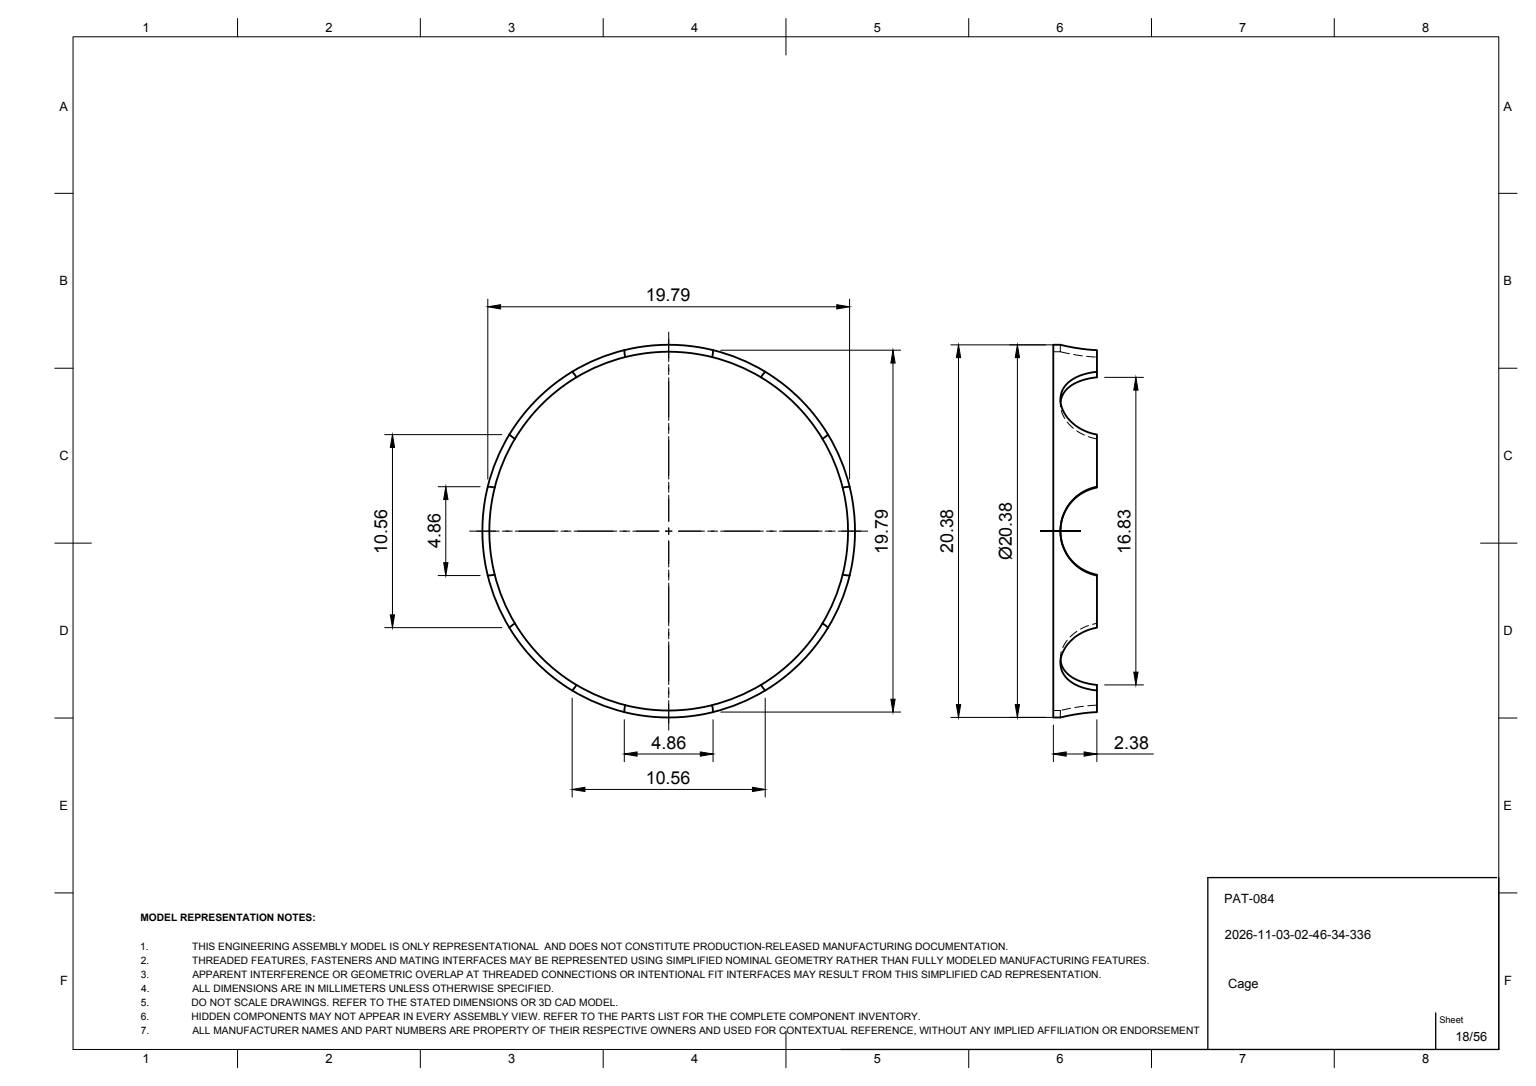
ISO-10303-21;
HEADER;
/* Generated by software containing ST-Developer
 * from STEP Tools, Inc. (www.steptools.com) 
 */

FILE_DESCRIPTION(
/* description */ ('Quick-return (Whitworth) mechanism'),
/* implementation_level */ '2;1');

FILE_NAME(
/* name */ 'Cage.step',
/* time_stamp */ '2026-10-28T03:25:57-07:00',
/* author */ (''),
/* organization */ (''),
/* preprocessor_version */ 'ST-DEVELOPER v20.2',
/* originating_system */ 'Autodesk Translation Framework v15.17.0.0',
/* authorisation */ '');

FILE_SCHEMA (('AUTOMOTIVE_DESIGN { 1 0 10303 214 3 1 1 }'));
ENDSEC;

DATA;
#10=MECHANICAL_DESIGN_GEOMETRIC_PRESENTATION_REPRESENTATION('',(#508),#14878);
#341=SPHERICAL_SURFACE('',#8767,0.247676);
#342=SPHERICAL_SURFACE('',#8783,0.247676);
#343=SPHERICAL_SURFACE('',#8788,0.247676);
#344=SPHERICAL_SURFACE('',#8793,0.247676);
#345=SPHERICAL_SURFACE('',#8798,0.247676);
#346=SPHERICAL_SURFACE('',#8803,0.247676);
#347=SPHERICAL_SURFACE('',#8808,0.247676);
#348=SPHERICAL_SURFACE('',#8816,0.247676);
#374=B_SPLINE_CURVE_WITH_KNOTS('',3,(#12898,#12899,#12900,#12901,#12902,
#12903,#12904,#12905,#12906,#12907,#12908,#12909,#12910,#12911,#12912,#12913,
#12914,#12915,#12916,#12917,#12918,#12919),.UNSPECIFIED.,.F.,.F.,(4,2,2,
2,2,2,2,2,2,2,4),(0.0473477652366656,0.126350602536658,0.189525903804987,
0.252701205073317,0.313298422430275,0.373895639787233,0.434492857144191,
0.495090074501149,0.558265375769478,0.621440677037807,0.7004435143378),
 .UNSPECIFIED.);
#375=B_SPLINE_CURVE_WITH_KNOTS('',3,(#12923,#12924,#12925,#12926,#12927,
#12928,#12929,#12930,#12931,#12932,#12933,#12934,#12935,#12936,#12937,#12938,
#12939,#12940,#12941,#12942,#12943,#12944),.UNSPECIFIED.,.F.,.F.,(4,2,2,
2,2,2,2,2,2,2,4),(0.0464897534940957,0.0852567806515119,0.170513561303024,
0.246687263103517,0.308657850341199,0.370628437578881,0.432599024816563,
0.494569612054245,0.570743313854739,0.656000094506251,0.694767121663666),
 .UNSPECIFIED.);
#376=B_SPLINE_CURVE_WITH_KNOTS('',3,(#12950,#12951,#12952,#12953,#12954,
#12955,#12956,#12957,#12958,#12959,#12960,#12961,#12962,#12963,#12964,#12965,
#12966,#12967,#12968,#12969,#12970,#12971),.UNSPECIFIED.,.F.,.F.,(4,2,2,
2,2,2,2,2,2,2,4),(0.0464897534940957,0.0852567806515118,0.170513561303024,
0.246687263103517,0.308657850341199,0.370628437578881,0.432599024816563,
0.494569612054245,0.570743313854738,0.65600009450625,0.694767121663666),
 .UNSPECIFIED.);
#377=B_SPLINE_CURVE_WITH_KNOTS('',3,(#12975,#12976,#12977,#12978,#12979,
#12980,#12981,#12982,#12983,#12984,#12985,#12986,#12987,#12988,#12989,#12990,
#12991,#12992,#12993,#12994,#12995,#12996),.UNSPECIFIED.,.F.,.F.,(4,2,2,
2,2,2,2,2,2,2,4),(0.0464897534940957,0.0852567806515119,0.170513561303024,
0.246687263103517,0.308657850341199,0.370628437578881,0.432599024816563,
0.494569612054245,0.570743313854739,0.656000094506251,0.694767121663666),
 .UNSPECIFIED.);
#378=B_SPLINE_CURVE_WITH_KNOTS('',3,(#13000,#13001,#13002,#13003,#13004,
#13005,#13006,#13007,#13008,#13009,#13010,#13011),.UNSPECIFIED.,.F.,.F.,
(4,2,2,2,2,4),(0.0464897534940957,0.0852567806515119,0.170513561303024,
0.246687263103517,0.308657850341199,0.370628437578881),.UNSPECIFIED.);
#379=B_SPLINE_CURVE_WITH_KNOTS('',3,(#13016,#13017,#13018,#13019,#13020,
#13021,#13022,#13023,#13024,#13025,#13026,#13027),.UNSPECIFIED.,.F.,.F.,
(4,2,2,2,2,4),(0.370628437578881,0.432599024816563,0.494569612054245,0.570743313854738,
0.65600009450625,0.694767121663666),.UNSPECIFIED.);
#380=B_SPLINE_CURVE_WITH_KNOTS('',3,(#13031,#13032,#13033,#13034,#13035,
#13036,#13037,#13038,#13039,#13040,#13041,#13042,#13043,#13044,#13045,#13046,
#13047,#13048,#13049,#13050,#13051,#13052),.UNSPECIFIED.,.F.,.F.,(4,2,2,
2,2,2,2,2,2,2,4),(0.0464897534940957,0.0852567806515121,0.170513561303024,
0.246687263103518,0.308657850341199,0.370628437578881,0.432599024816563,
0.494569612054245,0.570743313854738,0.65600009450625,0.694767121663666),
 .UNSPECIFIED.);
#381=B_SPLINE_CURVE_WITH_KNOTS('',3,(#13056,#13057,#13058,#13059,#13060,
#13061,#13062,#13063,#13064,#13065,#13066,#13067,#13068,#13069,#13070,#13071,
#13072,#13073,#13074,#13075,#13076,#13077),.UNSPECIFIED.,.F.,.F.,(4,2,2,
2,2,2,2,2,2,2,4),(0.0464897534940957,0.0852567806515119,0.170513561303024,
0.246687263103517,0.308657850341199,0.370628437578881,0.432599024816563,
0.494569612054245,0.570743313854738,0.65600009450625,0.694767121663667),
 .UNSPECIFIED.);
#382=B_SPLINE_CURVE_WITH_KNOTS('',3,(#13081,#13082,#13083,#13084,#13085,
#13086,#13087,#13088,#13089,#13090,#13091,#13092,#13093,#13094,#13095,#13096,
#13097,#13098,#13099,#13100,#13101,#13102),.UNSPECIFIED.,.F.,.F.,(4,2,2,
2,2,2,2,2,2,2,4),(0.0464897534940957,0.0852567806515119,0.170513561303024,
0.246687263103517,0.308657850341199,0.370628437578881,0.432599024816563,
0.494569612054245,0.570743313854738,0.65600009450625,0.694767121663666),
 .UNSPECIFIED.);
#383=B_SPLINE_CURVE_WITH_KNOTS('',3,(#13106,#13107,#13108,#13109,#13110,
#13111,#13112,#13113,#13114,#13115,#13116,#13117,#13118,#13119,#13120,#13121,
#13122,#13123,#13124,#13125,#13126,#13127),.UNSPECIFIED.,.F.,.F.,(4,2,2,
2,2,2,2,2,2,2,4),(0.0464897534940957,0.0852567806515119,0.170513561303024,
0.246687263103517,0.308657850341199,0.370628437578881,0.432599024816563,
0.494569612054245,0.570743313854739,0.656000094506251,0.694767121663667),
 .UNSPECIFIED.);
#384=B_SPLINE_CURVE_WITH_KNOTS('',3,(#13135,#13136,#13137,#13138,#13139,
#13140,#13141,#13142,#13143,#13144,#13145,#13146,#13147,#13148,#13149,#13150,
#13151,#13152,#13153,#13154,#13155,#13156),.UNSPECIFIED.,.F.,.F.,(4,2,2,
2,2,2,2,2,2,2,4),(0.0473477652366656,0.126350602536658,0.189525903804987,
0.252701205073316,0.313298422430274,0.373895639787232,0.434492857144191,
0.495090074501149,0.558265375769478,0.621440677037807,0.7004435143378),
 .UNSPECIFIED.);
#385=B_SPLINE_CURVE_WITH_KNOTS('',3,(#13164,#13165,#13166,#13167,#13168,
#13169,#13170,#13171,#13172,#13173,#13174,#13175,#13176,#13177,#13178,#13179,
#13180,#13181,#13182,#13183,#13184,#13185),.UNSPECIFIED.,.F.,.F.,(4,2,2,
2,2,2,2,2,2,2,4),(0.0473477652366656,0.126350602536658,0.189525903804987,
0.252701205073317,0.313298422430275,0.373895639787233,0.434492857144191,
0.495090074501149,0.558265375769478,0.621440677037807,0.7004435143378),
 .UNSPECIFIED.);
#386=B_SPLINE_CURVE_WITH_KNOTS('',3,(#13194,#13195,#13196,#13197,#13198,
#13199,#13200,#13201,#13202,#13203,#13204,#13205),.UNSPECIFIED.,.F.,.F.,
(4,2,2,2,2,4),(0.0473477652366656,0.126350602536658,0.189525903804987,0.252701205073316,
0.313298422430275,0.373895639787233),.UNSPECIFIED.);
#387=B_SPLINE_CURVE_WITH_KNOTS('',3,(#13207,#13208,#13209,#13210,#13211,
#13212,#13213,#13214,#13215,#13216,#13217,#13218),.UNSPECIFIED.,.F.,.F.,
(4,2,2,2,2,4),(0.373895639787233,0.434492857144191,0.495090074501149,0.558265375769478,
0.621440677037807,0.7004435143378),.UNSPECIFIED.);
#388=B_SPLINE_CURVE_WITH_KNOTS('',3,(#13225,#13226,#13227,#13228,#13229,
#13230,#13231,#13232,#13233,#13234,#13235,#13236,#13237,#13238,#13239,#13240,
#13241,#13242,#13243,#13244,#13245,#13246),.UNSPECIFIED.,.F.,.F.,(4,2,2,
2,2,2,2,2,2,2,4),(0.0473477652366656,0.126350602536658,0.189525903804987,
0.252701205073316,0.313298422430275,0.373895639787233,0.434492857144191,
0.495090074501149,0.558265375769478,0.621440677037807,0.7004435143378),
 .UNSPECIFIED.);
#389=B_SPLINE_CURVE_WITH_KNOTS('',3,(#13254,#13255,#13256,#13257,#13258,
#13259,#13260,#13261,#13262,#13263,#13264,#13265,#13266,#13267,#13268,#13269,
#13270,#13271,#13272,#13273,#13274,#13275),.UNSPECIFIED.,.F.,.F.,(4,2,2,
2,2,2,2,2,2,2,4),(0.0473477652366656,0.126350602536658,0.189525903804987,
0.252701205073317,0.313298422430275,0.373895639787233,0.434492857144191,
0.495090074501149,0.558265375769478,0.621440677037807,0.7004435143378),
 .UNSPECIFIED.);
#390=B_SPLINE_CURVE_WITH_KNOTS('',3,(#13283,#13284,#13285,#13286,#13287,
#13288,#13289,#13290,#13291,#13292,#13293,#13294,#13295,#13296,#13297,#13298,
#13299,#13300,#13301,#13302,#13303,#13304),.UNSPECIFIED.,.F.,.F.,(4,2,2,
2,2,2,2,2,2,2,4),(0.0473477652366656,0.126350602536658,0.189525903804987,
0.252701205073316,0.313298422430275,0.373895639787233,0.434492857144191,
0.495090074501149,0.558265375769478,0.621440677037807,0.7004435143378),
 .UNSPECIFIED.);
#391=B_SPLINE_CURVE_WITH_KNOTS('',3,(#13313,#13314,#13315,#13316,#13317,
#13318,#13319,#13320,#13321,#13322,#13323,#13324,#13325,#13326,#13327,#13328,
#13329,#13330,#13331,#13332,#13333,#13334),.UNSPECIFIED.,.F.,.F.,(4,2,2,
2,2,2,2,2,2,2,4),(0.0473477652366656,0.126350602536658,0.189525903804987,
0.252701205073317,0.313298422430275,0.373895639787233,0.434492857144191,
0.495090074501149,0.558265375769478,0.621440677037807,0.7004435143378),
 .UNSPECIFIED.);
#413=SHAPE_REPRESENTATION_RELATIONSHIP('SRR','None',#15082,#457);
#457=ADVANCED_BREP_SHAPE_REPRESENTATION('',(#560),#14839);
#508=STYLED_ITEM('',(#15406),#560);
#560=MANIFOLD_SOLID_BREP('Continuous crown cage',#7862);
#697=FACE_BOUND('',#1811,.T.);
#860=PLANE('',#8780);
#861=PLANE('',#8785);
#862=PLANE('',#8790);
#863=PLANE('',#8795);
#864=PLANE('',#8800);
#865=PLANE('',#8805);
#866=PLANE('',#8814);
#867=PLANE('',#8818);
#868=PLANE('',#8819);
#1221=FACE_OUTER_BOUND('',#1793,.T.);
#1222=FACE_OUTER_BOUND('',#1794,.T.);
#1223=FACE_OUTER_BOUND('',#1795,.T.);
#1224=FACE_OUTER_BOUND('',#1796,.T.);
#1225=FACE_OUTER_BOUND('',#1797,.T.);
#1226=FACE_OUTER_BOUND('',#1798,.T.);
#1227=FACE_OUTER_BOUND('',#1799,.T.);
#1228=FACE_OUTER_BOUND('',#1800,.T.);
#1229=FACE_OUTER_BOUND('',#1801,.T.);
#1230=FACE_OUTER_BOUND('',#1802,.T.);
#1231=FACE_OUTER_BOUND('',#1803,.T.);
#1232=FACE_OUTER_BOUND('',#1804,.T.);
#1233=FACE_OUTER_BOUND('',#1805,.T.);
#1234=FACE_OUTER_BOUND('',#1806,.T.);
#1235=FACE_OUTER_BOUND('',#1807,.T.);
#1236=FACE_OUTER_BOUND('',#1808,.T.);
#1237=FACE_OUTER_BOUND('',#1809,.T.);
#1238=FACE_OUTER_BOUND('',#1810,.T.);
#1239=FACE_OUTER_BOUND('',#1812,.T.);
#1793=EDGE_LOOP('',(#5998,#5999,#6000,#6001));
#1794=EDGE_LOOP('',(#6002,#6003,#6004,#6005,#6006,#6007,#6008,#6009,#6010,
#6011,#6012,#6013,#6014,#6015,#6016,#6017,#6018,#6019,#6020,#6021));
#1795=EDGE_LOOP('',(#6022,#6023,#6024,#6025));
#1796=EDGE_LOOP('',(#6026,#6027,#6028,#6029));
#1797=EDGE_LOOP('',(#6030,#6031,#6032,#6033));
#1798=EDGE_LOOP('',(#6034,#6035,#6036,#6037));
#1799=EDGE_LOOP('',(#6038,#6039,#6040,#6041));
#1800=EDGE_LOOP('',(#6042,#6043,#6044,#6045,#6046,#6047));
#1801=EDGE_LOOP('',(#6048,#6049,#6050,#6051));
#1802=EDGE_LOOP('',(#6052,#6053,#6054,#6055));
#1803=EDGE_LOOP('',(#6056,#6057,#6058,#6059));
#1804=EDGE_LOOP('',(#6060,#6061,#6062,#6063));
#1805=EDGE_LOOP('',(#6064,#6065,#6066,#6067));
#1806=EDGE_LOOP('',(#6068,#6069,#6070,#6071));
#1807=EDGE_LOOP('',(#6072,#6073,#6074,#6075,#6076,#6077,#6078,#6079,#6080,
#6081,#6082,#6083,#6084,#6085,#6086,#6087,#6088,#6089,#6090,#6091));
#1808=EDGE_LOOP('',(#6092,#6093,#6094,#6095));
#1809=EDGE_LOOP('',(#6096,#6097,#6098,#6099));
#1810=EDGE_LOOP('',(#6100));
#1811=EDGE_LOOP('',(#6101));
#1812=EDGE_LOOP('',(#6102,#6103,#6104,#6105));
#2336=LINE('',#13013,#2859);
#2337=LINE('',#13309,#2860);
#2859=VECTOR('',#10343,1.019052);
#2860=VECTOR('',#10420,0.980948);
#3410=CIRCLE('',#8768,0.243053047864041);
#3411=CIRCLE('',#8769,0.243053047864041);
#3412=CIRCLE('',#8771,1.019052);
#3413=CIRCLE('',#8772,1.019052);
#3414=CIRCLE('',#8773,1.019052);
#3415=CIRCLE('',#8774,1.019052);
#3416=CIRCLE('',#8775,1.019052);
#3417=CIRCLE('',#8776,1.019052);
#3418=CIRCLE('',#8777,1.019052);
#3419=CIRCLE('',#8778,1.019052);
#3420=CIRCLE('',#8779,1.019052);
#3421=CIRCLE('',#8781,0.980948);
#3422=CIRCLE('',#8782,0.243053047864041);
#3423=CIRCLE('',#8784,0.243053047864041);
#3424=CIRCLE('',#8786,0.980948);
#3425=CIRCLE('',#8787,0.243053047864041);
#3426=CIRCLE('',#8789,0.243053047864041);
#3427=CIRCLE('',#8791,0.980948);
#3428=CIRCLE('',#8792,0.243053047864041);
#3429=CIRCLE('',#8794,0.243053047864041);
#3430=CIRCLE('',#8796,0.980948);
#3431=CIRCLE('',#8797,0.243053047864041);
#3432=CIRCLE('',#8799,0.243053047864041);
#3433=CIRCLE('',#8801,0.980948);
#3434=CIRCLE('',#8802,0.243053047864041);
#3435=CIRCLE('',#8804,0.243053047864041);
#3436=CIRCLE('',#8806,0.980948);
#3437=CIRCLE('',#8807,0.243053047864041);
#3438=CIRCLE('',#8809,0.243053047864041);
#3439=CIRCLE('',#8811,0.980948);
#3440=CIRCLE('',#8812,0.980948);
#3441=CIRCLE('',#8813,0.980948);
#3442=CIRCLE('',#8815,0.243053047864041);
#3443=CIRCLE('',#8817,0.243053047864041);
#3887=VERTEX_POINT('',#12896);
#3888=VERTEX_POINT('',#12897);
#3889=VERTEX_POINT('',#12920);
#3890=VERTEX_POINT('',#12922);
#3891=VERTEX_POINT('',#12947);
#3892=VERTEX_POINT('',#12949);
#3893=VERTEX_POINT('',#12972);
#3894=VERTEX_POINT('',#12974);
#3895=VERTEX_POINT('',#12997);
#3896=VERTEX_POINT('',#12999);
#3897=VERTEX_POINT('',#13012);
#3898=VERTEX_POINT('',#13015);
#3899=VERTEX_POINT('',#13028);
#3900=VERTEX_POINT('',#13030);
#3901=VERTEX_POINT('',#13053);
#3902=VERTEX_POINT('',#13055);
#3903=VERTEX_POINT('',#13078);
#3904=VERTEX_POINT('',#13080);
#3905=VERTEX_POINT('',#13103);
#3906=VERTEX_POINT('',#13105);
#3907=VERTEX_POINT('',#13130);
#3908=VERTEX_POINT('',#13134);
#3909=VERTEX_POINT('',#13159);
#3910=VERTEX_POINT('',#13163);
#3911=VERTEX_POINT('',#13188);
#3912=VERTEX_POINT('',#13192);
#3913=VERTEX_POINT('',#13193);
#3914=VERTEX_POINT('',#13220);
#3915=VERTEX_POINT('',#13224);
#3916=VERTEX_POINT('',#13249);
#3917=VERTEX_POINT('',#13253);
#3918=VERTEX_POINT('',#13278);
#3919=VERTEX_POINT('',#13282);
#3920=VERTEX_POINT('',#13307);
#3921=VERTEX_POINT('',#13310);
#3922=VERTEX_POINT('',#13312);
#4656=EDGE_CURVE('',#3887,#3888,#374,.T.);
#4657=EDGE_CURVE('',#3889,#3887,#3410,.T.);
#4658=EDGE_CURVE('',#3890,#3889,#375,.T.);
#4659=EDGE_CURVE('',#3888,#3890,#3411,.T.);
#4660=EDGE_CURVE('',#3891,#3889,#3412,.T.);
#4661=EDGE_CURVE('',#3891,#3892,#376,.T.);
#4662=EDGE_CURVE('',#3893,#3892,#3413,.T.);
#4663=EDGE_CURVE('',#3893,#3894,#377,.T.);
#4664=EDGE_CURVE('',#3895,#3894,#3414,.T.);
#4665=EDGE_CURVE('',#3895,#3896,#378,.T.);
#4666=EDGE_CURVE('',#3896,#3897,#2336,.T.);
#4667=EDGE_CURVE('',#3897,#3897,#3415,.T.);
#4668=EDGE_CURVE('',#3896,#3898,#379,.T.);
#4669=EDGE_CURVE('',#3899,#3898,#3416,.T.);
#4670=EDGE_CURVE('',#3899,#3900,#380,.T.);
#4671=EDGE_CURVE('',#3901,#3900,#3417,.T.);
#4672=EDGE_CURVE('',#3901,#3902,#381,.T.);
#4673=EDGE_CURVE('',#3903,#3902,#3418,.T.);
#4674=EDGE_CURVE('',#3903,#3904,#382,.T.);
#4675=EDGE_CURVE('',#3905,#3904,#3419,.T.);
#4676=EDGE_CURVE('',#3905,#3906,#383,.T.);
#4677=EDGE_CURVE('',#3890,#3906,#3420,.T.);
#4678=EDGE_CURVE('',#3887,#3907,#3421,.T.);
#4679=EDGE_CURVE('',#3907,#3891,#3422,.T.);
#4680=EDGE_CURVE('',#3908,#3907,#384,.T.);
#4681=EDGE_CURVE('',#3892,#3908,#3423,.T.);
#4682=EDGE_CURVE('',#3908,#3909,#3424,.T.);
#4683=EDGE_CURVE('',#3909,#3893,#3425,.T.);
#4684=EDGE_CURVE('',#3910,#3909,#385,.T.);
#4685=EDGE_CURVE('',#3894,#3910,#3426,.T.);
#4686=EDGE_CURVE('',#3910,#3911,#3427,.T.);
#4687=EDGE_CURVE('',#3911,#3895,#3428,.T.);
#4688=EDGE_CURVE('',#3912,#3913,#386,.T.);
#4689=EDGE_CURVE('',#3898,#3912,#3429,.T.);
#4690=EDGE_CURVE('',#3913,#3911,#387,.T.);
#4691=EDGE_CURVE('',#3912,#3914,#3430,.T.);
#4692=EDGE_CURVE('',#3914,#3899,#3431,.T.);
#4693=EDGE_CURVE('',#3915,#3914,#388,.T.);
#4694=EDGE_CURVE('',#3900,#3915,#3432,.T.);
#4695=EDGE_CURVE('',#3915,#3916,#3433,.T.);
#4696=EDGE_CURVE('',#3916,#3901,#3434,.T.);
#4697=EDGE_CURVE('',#3917,#3916,#389,.T.);
#4698=EDGE_CURVE('',#3902,#3917,#3435,.T.);
#4699=EDGE_CURVE('',#3917,#3918,#3436,.T.);
#4700=EDGE_CURVE('',#3918,#3903,#3437,.T.);
#4701=EDGE_CURVE('',#3919,#3918,#390,.T.);
#4702=EDGE_CURVE('',#3904,#3919,#3438,.T.);
#4703=EDGE_CURVE('',#3920,#3920,#3439,.T.);
#4704=EDGE_CURVE('',#3920,#3913,#2337,.T.);
#4705=EDGE_CURVE('',#3921,#3888,#3440,.T.);
#4706=EDGE_CURVE('',#3921,#3922,#391,.T.);
#4707=EDGE_CURVE('',#3919,#3922,#3441,.T.);
#4708=EDGE_CURVE('',#3906,#3921,#3442,.T.);
#4709=EDGE_CURVE('',#3922,#3905,#3443,.T.);
#5998=ORIENTED_EDGE('',*,*,#4656,.F.);
#5999=ORIENTED_EDGE('',*,*,#4657,.F.);
#6000=ORIENTED_EDGE('',*,*,#4658,.F.);
#6001=ORIENTED_EDGE('',*,*,#4659,.F.);
#6002=ORIENTED_EDGE('',*,*,#4658,.T.);
#6003=ORIENTED_EDGE('',*,*,#4660,.F.);
#6004=ORIENTED_EDGE('',*,*,#4661,.T.);
#6005=ORIENTED_EDGE('',*,*,#4662,.F.);
#6006=ORIENTED_EDGE('',*,*,#4663,.T.);
#6007=ORIENTED_EDGE('',*,*,#4664,.F.);
#6008=ORIENTED_EDGE('',*,*,#4665,.T.);
#6009=ORIENTED_EDGE('',*,*,#4666,.T.);
#6010=ORIENTED_EDGE('',*,*,#4667,.F.);
#6011=ORIENTED_EDGE('',*,*,#4666,.F.);
#6012=ORIENTED_EDGE('',*,*,#4668,.T.);
#6013=ORIENTED_EDGE('',*,*,#4669,.F.);
#6014=ORIENTED_EDGE('',*,*,#4670,.T.);
#6015=ORIENTED_EDGE('',*,*,#4671,.F.);
#6016=ORIENTED_EDGE('',*,*,#4672,.T.);
#6017=ORIENTED_EDGE('',*,*,#4673,.F.);
#6018=ORIENTED_EDGE('',*,*,#4674,.T.);
#6019=ORIENTED_EDGE('',*,*,#4675,.F.);
#6020=ORIENTED_EDGE('',*,*,#4676,.T.);
#6021=ORIENTED_EDGE('',*,*,#4677,.F.);
#6022=ORIENTED_EDGE('',*,*,#4657,.T.);
#6023=ORIENTED_EDGE('',*,*,#4678,.T.);
#6024=ORIENTED_EDGE('',*,*,#4679,.T.);
#6025=ORIENTED_EDGE('',*,*,#4660,.T.);
#6026=ORIENTED_EDGE('',*,*,#4680,.F.);
#6027=ORIENTED_EDGE('',*,*,#4681,.F.);
#6028=ORIENTED_EDGE('',*,*,#4661,.F.);
#6029=ORIENTED_EDGE('',*,*,#4679,.F.);
#6030=ORIENTED_EDGE('',*,*,#4681,.T.);
#6031=ORIENTED_EDGE('',*,*,#4682,.T.);
#6032=ORIENTED_EDGE('',*,*,#4683,.T.);
#6033=ORIENTED_EDGE('',*,*,#4662,.T.);
#6034=ORIENTED_EDGE('',*,*,#4684,.F.);
#6035=ORIENTED_EDGE('',*,*,#4685,.F.);
#6036=ORIENTED_EDGE('',*,*,#4663,.F.);
#6037=ORIENTED_EDGE('',*,*,#4683,.F.);
#6038=ORIENTED_EDGE('',*,*,#4685,.T.);
#6039=ORIENTED_EDGE('',*,*,#4686,.T.);
#6040=ORIENTED_EDGE('',*,*,#4687,.T.);
#6041=ORIENTED_EDGE('',*,*,#4664,.T.);
#6042=ORIENTED_EDGE('',*,*,#4688,.F.);
#6043=ORIENTED_EDGE('',*,*,#4689,.F.);
#6044=ORIENTED_EDGE('',*,*,#4668,.F.);
#6045=ORIENTED_EDGE('',*,*,#4665,.F.);
#6046=ORIENTED_EDGE('',*,*,#4687,.F.);
#6047=ORIENTED_EDGE('',*,*,#4690,.F.);
#6048=ORIENTED_EDGE('',*,*,#4689,.T.);
#6049=ORIENTED_EDGE('',*,*,#4691,.T.);
#6050=ORIENTED_EDGE('',*,*,#4692,.T.);
#6051=ORIENTED_EDGE('',*,*,#4669,.T.);
#6052=ORIENTED_EDGE('',*,*,#4693,.F.);
#6053=ORIENTED_EDGE('',*,*,#4694,.F.);
#6054=ORIENTED_EDGE('',*,*,#4670,.F.);
#6055=ORIENTED_EDGE('',*,*,#4692,.F.);
#6056=ORIENTED_EDGE('',*,*,#4694,.T.);
#6057=ORIENTED_EDGE('',*,*,#4695,.T.);
#6058=ORIENTED_EDGE('',*,*,#4696,.T.);
#6059=ORIENTED_EDGE('',*,*,#4671,.T.);
#6060=ORIENTED_EDGE('',*,*,#4697,.F.);
#6061=ORIENTED_EDGE('',*,*,#4698,.F.);
#6062=ORIENTED_EDGE('',*,*,#4672,.F.);
#6063=ORIENTED_EDGE('',*,*,#4696,.F.);
#6064=ORIENTED_EDGE('',*,*,#4698,.T.);
#6065=ORIENTED_EDGE('',*,*,#4699,.T.);
#6066=ORIENTED_EDGE('',*,*,#4700,.T.);
#6067=ORIENTED_EDGE('',*,*,#4673,.T.);
#6068=ORIENTED_EDGE('',*,*,#4674,.F.);
#6069=ORIENTED_EDGE('',*,*,#4700,.F.);
#6070=ORIENTED_EDGE('',*,*,#4701,.F.);
#6071=ORIENTED_EDGE('',*,*,#4702,.F.);
#6072=ORIENTED_EDGE('',*,*,#4703,.F.);
#6073=ORIENTED_EDGE('',*,*,#4704,.T.);
#6074=ORIENTED_EDGE('',*,*,#4690,.T.);
#6075=ORIENTED_EDGE('',*,*,#4686,.F.);
#6076=ORIENTED_EDGE('',*,*,#4684,.T.);
#6077=ORIENTED_EDGE('',*,*,#4682,.F.);
#6078=ORIENTED_EDGE('',*,*,#4680,.T.);
#6079=ORIENTED_EDGE('',*,*,#4678,.F.);
#6080=ORIENTED_EDGE('',*,*,#4656,.T.);
#6081=ORIENTED_EDGE('',*,*,#4705,.F.);
#6082=ORIENTED_EDGE('',*,*,#4706,.T.);
#6083=ORIENTED_EDGE('',*,*,#4707,.F.);
#6084=ORIENTED_EDGE('',*,*,#4701,.T.);
#6085=ORIENTED_EDGE('',*,*,#4699,.F.);
#6086=ORIENTED_EDGE('',*,*,#4697,.T.);
#6087=ORIENTED_EDGE('',*,*,#4695,.F.);
#6088=ORIENTED_EDGE('',*,*,#4693,.T.);
#6089=ORIENTED_EDGE('',*,*,#4691,.F.);
#6090=ORIENTED_EDGE('',*,*,#4688,.T.);
#6091=ORIENTED_EDGE('',*,*,#4704,.F.);
#6092=ORIENTED_EDGE('',*,*,#4659,.T.);
#6093=ORIENTED_EDGE('',*,*,#4677,.T.);
#6094=ORIENTED_EDGE('',*,*,#4708,.T.);
#6095=ORIENTED_EDGE('',*,*,#4705,.T.);
#6096=ORIENTED_EDGE('',*,*,#4676,.F.);
#6097=ORIENTED_EDGE('',*,*,#4709,.F.);
#6098=ORIENTED_EDGE('',*,*,#4706,.F.);
#6099=ORIENTED_EDGE('',*,*,#4708,.F.);
#6100=ORIENTED_EDGE('',*,*,#4667,.T.);
#6101=ORIENTED_EDGE('',*,*,#4703,.T.);
#6102=ORIENTED_EDGE('',*,*,#4702,.T.);
#6103=ORIENTED_EDGE('',*,*,#4707,.T.);
#6104=ORIENTED_EDGE('',*,*,#4709,.T.);
#6105=ORIENTED_EDGE('',*,*,#4675,.T.);
#7292=CYLINDRICAL_SURFACE('',#8770,1.019052);
#7293=CYLINDRICAL_SURFACE('',#8810,0.980948);
#7552=ADVANCED_FACE('',(#1221),#341,.F.);
#7553=ADVANCED_FACE('',(#1222),#7292,.T.);
#7554=ADVANCED_FACE('',(#1223),#860,.T.);
#7555=ADVANCED_FACE('',(#1224),#342,.F.);
#7556=ADVANCED_FACE('',(#1225),#861,.T.);
#7557=ADVANCED_FACE('',(#1226),#343,.F.);
#7558=ADVANCED_FACE('',(#1227),#862,.T.);
#7559=ADVANCED_FACE('',(#1228),#344,.F.);
#7560=ADVANCED_FACE('',(#1229),#863,.T.);
#7561=ADVANCED_FACE('',(#1230),#345,.F.);
#7562=ADVANCED_FACE('',(#1231),#864,.T.);
#7563=ADVANCED_FACE('',(#1232),#346,.F.);
#7564=ADVANCED_FACE('',(#1233),#865,.T.);
#7565=ADVANCED_FACE('',(#1234),#347,.F.);
#7566=ADVANCED_FACE('',(#1235),#7293,.F.);
#7567=ADVANCED_FACE('',(#1236),#866,.T.);
#7568=ADVANCED_FACE('',(#1237),#348,.F.);
#7569=ADVANCED_FACE('',(#1238,#697),#867,.T.);
#7570=ADVANCED_FACE('',(#1239),#868,.T.);
#7862=CLOSED_SHELL('',(#7552,#7553,#7554,#7555,#7556,#7557,#7558,#7559,
#7560,#7561,#7562,#7563,#7564,#7565,#7566,#7567,#7568,#7569,#7570));
#8766=AXIS2_PLACEMENT_3D('',#12894,#10327,#10328);
#8767=AXIS2_PLACEMENT_3D('',#12895,#10329,#10330);
#8768=AXIS2_PLACEMENT_3D('',#12921,#10331,#10332);
#8769=AXIS2_PLACEMENT_3D('',#12945,#10333,#10334);
#8770=AXIS2_PLACEMENT_3D('',#12946,#10335,#10336);
#8771=AXIS2_PLACEMENT_3D('',#12948,#10337,#10338);
#8772=AXIS2_PLACEMENT_3D('',#12973,#10339,#10340);
#8773=AXIS2_PLACEMENT_3D('',#12998,#10341,#10342);
#8774=AXIS2_PLACEMENT_3D('',#13014,#10344,#10345);
#8775=AXIS2_PLACEMENT_3D('',#13029,#10346,#10347);
#8776=AXIS2_PLACEMENT_3D('',#13054,#10348,#10349);
#8777=AXIS2_PLACEMENT_3D('',#13079,#10350,#10351);
#8778=AXIS2_PLACEMENT_3D('',#13104,#10352,#10353);
#8779=AXIS2_PLACEMENT_3D('',#13128,#10354,#10355);
#8780=AXIS2_PLACEMENT_3D('',#13129,#10356,#10357);
#8781=AXIS2_PLACEMENT_3D('',#13131,#10358,#10359);
#8782=AXIS2_PLACEMENT_3D('',#13132,#10360,#10361);
#8783=AXIS2_PLACEMENT_3D('',#13133,#10362,#10363);
#8784=AXIS2_PLACEMENT_3D('',#13157,#10364,#10365);
#8785=AXIS2_PLACEMENT_3D('',#13158,#10366,#10367);
#8786=AXIS2_PLACEMENT_3D('',#13160,#10368,#10369);
#8787=AXIS2_PLACEMENT_3D('',#13161,#10370,#10371);
#8788=AXIS2_PLACEMENT_3D('',#13162,#10372,#10373);
#8789=AXIS2_PLACEMENT_3D('',#13186,#10374,#10375);
#8790=AXIS2_PLACEMENT_3D('',#13187,#10376,#10377);
#8791=AXIS2_PLACEMENT_3D('',#13189,#10378,#10379);
#8792=AXIS2_PLACEMENT_3D('',#13190,#10380,#10381);
#8793=AXIS2_PLACEMENT_3D('',#13191,#10382,#10383);
#8794=AXIS2_PLACEMENT_3D('',#13206,#10384,#10385);
#8795=AXIS2_PLACEMENT_3D('',#13219,#10386,#10387);
#8796=AXIS2_PLACEMENT_3D('',#13221,#10388,#10389);
#8797=AXIS2_PLACEMENT_3D('',#13222,#10390,#10391);
#8798=AXIS2_PLACEMENT_3D('',#13223,#10392,#10393);
#8799=AXIS2_PLACEMENT_3D('',#13247,#10394,#10395);
#8800=AXIS2_PLACEMENT_3D('',#13248,#10396,#10397);
#8801=AXIS2_PLACEMENT_3D('',#13250,#10398,#10399);
#8802=AXIS2_PLACEMENT_3D('',#13251,#10400,#10401);
#8803=AXIS2_PLACEMENT_3D('',#13252,#10402,#10403);
#8804=AXIS2_PLACEMENT_3D('',#13276,#10404,#10405);
#8805=AXIS2_PLACEMENT_3D('',#13277,#10406,#10407);
#8806=AXIS2_PLACEMENT_3D('',#13279,#10408,#10409);
#8807=AXIS2_PLACEMENT_3D('',#13280,#10410,#10411);
#8808=AXIS2_PLACEMENT_3D('',#13281,#10412,#10413);
#8809=AXIS2_PLACEMENT_3D('',#13305,#10414,#10415);
#8810=AXIS2_PLACEMENT_3D('',#13306,#10416,#10417);
#8811=AXIS2_PLACEMENT_3D('',#13308,#10418,#10419);
#8812=AXIS2_PLACEMENT_3D('',#13311,#10421,#10422);
#8813=AXIS2_PLACEMENT_3D('',#13335,#10423,#10424);
#8814=AXIS2_PLACEMENT_3D('',#13336,#10425,#10426);
#8815=AXIS2_PLACEMENT_3D('',#13337,#10427,#10428);
#8816=AXIS2_PLACEMENT_3D('',#13338,#10429,#10430);
#8817=AXIS2_PLACEMENT_3D('',#13339,#10431,#10432);
#8818=AXIS2_PLACEMENT_3D('',#13340,#10433,#10434);
#8819=AXIS2_PLACEMENT_3D('',#13341,#10435,#10436);
#10327=DIRECTION('axis',(0.,0.,1.));
#10328=DIRECTION('refdir',(1.,0.,0.));
#10329=DIRECTION('center_axis',(0.,0.,1.));
#10330=DIRECTION('ref_axis',(1.,0.,0.));
#10331=DIRECTION('center_axis',(0.,-1.,0.));
#10332=DIRECTION('ref_axis',(0.,0.,-1.));
#10333=DIRECTION('center_axis',(0.,-1.,0.));
#10334=DIRECTION('ref_axis',(0.,0.,-1.));
#10335=DIRECTION('center_axis',(0.,1.,0.));
#10336=DIRECTION('ref_axis',(1.,0.,0.));
#10337=DIRECTION('center_axis',(0.,1.,0.));
#10338=DIRECTION('ref_axis',(1.,0.,0.));
#10339=DIRECTION('center_axis',(0.,1.,0.));
#10340=DIRECTION('ref_axis',(1.,0.,0.));
#10341=DIRECTION('center_axis',(0.,1.,0.));
#10342=DIRECTION('ref_axis',(1.,0.,0.));
#10343=DIRECTION('',(0.,-1.,0.));
#10344=DIRECTION('center_axis',(0.,-1.,0.));
#10345=DIRECTION('ref_axis',(1.,0.,0.));
#10346=DIRECTION('center_axis',(0.,1.,0.));
#10347=DIRECTION('ref_axis',(1.,0.,0.));
#10348=DIRECTION('center_axis',(0.,1.,0.));
#10349=DIRECTION('ref_axis',(1.,0.,0.));
#10350=DIRECTION('center_axis',(0.,1.,0.));
#10351=DIRECTION('ref_axis',(1.,0.,0.));
#10352=DIRECTION('center_axis',(0.,1.,0.));
#10353=DIRECTION('ref_axis',(1.,0.,0.));
#10354=DIRECTION('center_axis',(0.,1.,0.));
#10355=DIRECTION('ref_axis',(1.,0.,0.));
#10356=DIRECTION('center_axis',(0.,1.,0.));
#10357=DIRECTION('ref_axis',(1.,0.,0.));
#10358=DIRECTION('center_axis',(0.,-1.,0.));
#10359=DIRECTION('ref_axis',(1.,0.,0.));
#10360=DIRECTION('center_axis',(0.,-1.,0.));
#10361=DIRECTION('ref_axis',(0.,0.,-1.));
#10362=DIRECTION('center_axis',(6.12323399573677E-17,0.,1.));
#10363=DIRECTION('ref_axis',(1.,0.,0.));
#10364=DIRECTION('center_axis',(0.,-1.,0.));
#10365=DIRECTION('ref_axis',(0.,0.,-1.));
#10366=DIRECTION('center_axis',(0.,1.,0.));
#10367=DIRECTION('ref_axis',(1.,0.,0.));
#10368=DIRECTION('center_axis',(0.,-1.,0.));
#10369=DIRECTION('ref_axis',(1.,0.,0.));
#10370=DIRECTION('center_axis',(0.,-1.,0.));
#10371=DIRECTION('ref_axis',(0.,0.,-1.));
#10372=DIRECTION('center_axis',(0.,0.,1.));
#10373=DIRECTION('ref_axis',(1.,0.,0.));
#10374=DIRECTION('center_axis',(0.,-1.,0.));
#10375=DIRECTION('ref_axis',(0.,0.,-1.));
#10376=DIRECTION('center_axis',(0.,1.,0.));
#10377=DIRECTION('ref_axis',(1.,0.,0.));
#10378=DIRECTION('center_axis',(0.,-1.,0.));
#10379=DIRECTION('ref_axis',(1.,0.,0.));
#10380=DIRECTION('center_axis',(0.,-1.,0.));
#10381=DIRECTION('ref_axis',(0.,0.,-1.));
#10382=DIRECTION('center_axis',(0.,0.,1.));
#10383=DIRECTION('ref_axis',(1.,0.,0.));
#10384=DIRECTION('center_axis',(0.,-1.,0.));
#10385=DIRECTION('ref_axis',(0.,0.,-1.));
#10386=DIRECTION('center_axis',(0.,1.,0.));
#10387=DIRECTION('ref_axis',(1.,0.,0.));
#10388=DIRECTION('center_axis',(0.,-1.,0.));
#10389=DIRECTION('ref_axis',(1.,0.,0.));
#10390=DIRECTION('center_axis',(0.,-1.,0.));
#10391=DIRECTION('ref_axis',(0.,0.,-1.));
#10392=DIRECTION('center_axis',(0.,0.,1.));
#10393=DIRECTION('ref_axis',(1.,0.,0.));
#10394=DIRECTION('center_axis',(0.,-1.,0.));
#10395=DIRECTION('ref_axis',(0.,0.,-1.));
#10396=DIRECTION('center_axis',(0.,1.,0.));
#10397=DIRECTION('ref_axis',(1.,0.,0.));
#10398=DIRECTION('center_axis',(0.,-1.,0.));
#10399=DIRECTION('ref_axis',(1.,0.,0.));
#10400=DIRECTION('center_axis',(0.,-1.,0.));
#10401=DIRECTION('ref_axis',(0.,0.,-1.));
#10402=DIRECTION('center_axis',(6.12323399573676E-17,0.,1.));
#10403=DIRECTION('ref_axis',(1.,0.,0.));
#10404=DIRECTION('center_axis',(0.,-1.,0.));
#10405=DIRECTION('ref_axis',(0.,0.,-1.));
#10406=DIRECTION('center_axis',(0.,1.,0.));
#10407=DIRECTION('ref_axis',(1.,0.,0.));
#10408=DIRECTION('center_axis',(0.,-1.,0.));
#10409=DIRECTION('ref_axis',(1.,0.,0.));
#10410=DIRECTION('center_axis',(0.,-1.,0.));
#10411=DIRECTION('ref_axis',(0.,0.,-1.));
#10412=DIRECTION('center_axis',(0.,0.,1.));
#10413=DIRECTION('ref_axis',(1.,0.,0.));
#10414=DIRECTION('center_axis',(0.,-1.,0.));
#10415=DIRECTION('ref_axis',(0.,0.,-1.));
#10416=DIRECTION('center_axis',(0.,1.,0.));
#10417=DIRECTION('ref_axis',(1.,0.,0.));
#10418=DIRECTION('center_axis',(0.,1.,0.));
#10419=DIRECTION('ref_axis',(1.,0.,0.));
#10420=DIRECTION('',(0.,1.,0.));
#10421=DIRECTION('center_axis',(0.,-1.,0.));
#10422=DIRECTION('ref_axis',(1.,0.,0.));
#10423=DIRECTION('center_axis',(0.,-1.,0.));
#10424=DIRECTION('ref_axis',(1.,0.,0.));
#10425=DIRECTION('center_axis',(0.,1.,0.));
#10426=DIRECTION('ref_axis',(1.,0.,0.));
#10427=DIRECTION('center_axis',(0.,-1.,0.));
#10428=DIRECTION('ref_axis',(0.,0.,-1.));
#10429=DIRECTION('center_axis',(0.,0.,1.));
#10430=DIRECTION('ref_axis',(1.,0.,0.));
#10431=DIRECTION('center_axis',(0.,-1.,0.));
#10432=DIRECTION('ref_axis',(0.,0.,-1.));
#10433=DIRECTION('center_axis',(0.,-1.,0.));
#10434=DIRECTION('ref_axis',(-1.,0.,0.));
#10435=DIRECTION('center_axis',(0.,1.,0.));
#10436=DIRECTION('ref_axis',(1.,0.,0.));
#12894=CARTESIAN_POINT('',(0.,0.,0.));
#12895=CARTESIAN_POINT('Origin',(0.707106781186547,0.,0.707106781186548));
#12896=CARTESIAN_POINT('',(0.504455939115715,-0.04763,0.841298510752802));
#12897=CARTESIAN_POINT('',(0.841298510752802,-0.04763,0.504455939115715));
#12898=CARTESIAN_POINT('Ctrl Pts',(0.504455939115715,-0.04763,0.841298510752802));
#12899=CARTESIAN_POINT('Ctrl Pts',(0.508899795931835,-0.0740444353928835,
0.838633903678357));
#12900=CARTESIAN_POINT('Ctrl Pts',(0.517157748491652,-0.0999305678883309,
0.833661031856294));
#12901=CARTESIAN_POINT('Ctrl Pts',(0.537715343527944,-0.142345102874864,
0.820511285096538));
#12902=CARTESIAN_POINT('Ctrl Pts',(0.548874290046456,-0.159766064500479,
0.813159949759));
#12903=CARTESIAN_POINT('Ctrl Pts',(0.573915184558107,-0.190326085855194,
0.795684265985089));
#12904=CARTESIAN_POINT('Ctrl Pts',(0.587792702767295,-0.203463743702801,
0.78555112003688));
#12905=CARTESIAN_POINT('Ctrl Pts',(0.615966552324775,-0.224161999508995,
0.763642258217233));
#12906=CARTESIAN_POINT('Ctrl Pts',(0.631684198665438,-0.232861760990032,
0.750785745543687));
#12907=CARTESIAN_POINT('Ctrl Pts',(0.663382628119203,-0.244251601209411,
0.722929908501543));
#12908=CARTESIAN_POINT('Ctrl Pts',(0.679352081686668,-0.246942143572133,
0.707917883896095));
#12909=CARTESIAN_POINT('Ctrl Pts',(0.707917883896095,-0.246942143572133,
0.679352081686668));
#12910=CARTESIAN_POINT('Ctrl Pts',(0.722929908501543,-0.244251601209411,
0.663382628119203));
#12911=CARTESIAN_POINT('Ctrl Pts',(0.750785745543687,-0.232861760990032,
0.631684198665439));
#12912=CARTESIAN_POINT('Ctrl Pts',(0.763642258217232,-0.224161999508995,
0.615966552324775));
#12913=CARTESIAN_POINT('Ctrl Pts',(0.78555112003688,-0.203463743702801,
0.587792702767295));
#12914=CARTESIAN_POINT('Ctrl Pts',(0.795684265985088,-0.190326085855194,
0.573915184558108));
#12915=CARTESIAN_POINT('Ctrl Pts',(0.813159949759,-0.15976606450048,0.548874290046456));
#12916=CARTESIAN_POINT('Ctrl Pts',(0.820511285096538,-0.142345102874864,
0.537715343527944));
#12917=CARTESIAN_POINT('Ctrl Pts',(0.833661031856294,-0.099930567888331,
0.517157748491653));
#12918=CARTESIAN_POINT('Ctrl Pts',(0.838633903678357,-0.0740444353928835,
0.508899795931835));
#12919=CARTESIAN_POINT('Ctrl Pts',(0.841298510752801,-0.0476299999999999,
0.504455939115715));
#12920=CARTESIAN_POINT('',(0.528110872004958,-0.04763,0.871530771444223));
#12921=CARTESIAN_POINT('Origin',(0.707106781186547,-0.04763,0.707106781186548));
#12922=CARTESIAN_POINT('',(0.871530771444223,-0.04763,0.528110872004959));
#12923=CARTESIAN_POINT('Ctrl Pts',(0.871530771444223,-0.0476300000000001,
0.528110872004958));
#12924=CARTESIAN_POINT('Ctrl Pts',(0.87014664509073,-0.0609922781173483,
0.530395067942936));
#12925=CARTESIAN_POINT('Ctrl Pts',(0.868149331745851,-0.0742967091364493,
0.533674141594226));
#12926=CARTESIAN_POINT('Ctrl Pts',(0.85981294420286,-0.115492077056649,
0.54708917182331));
#12927=CARTESIAN_POINT('Ctrl Pts',(0.850993704737257,-0.141695629206859,
0.560922177770136));
#12928=CARTESIAN_POINT('Ctrl Pts',(0.830754510485543,-0.181890537957859,
0.590422647829571));
#12929=CARTESIAN_POINT('Ctrl Pts',(0.816896541396381,-0.201072148666545,
0.609616703125488));
#12930=CARTESIAN_POINT('Ctrl Pts',(0.792310597819928,-0.223955109275652,
0.641117951819998));
#12931=CARTESIAN_POINT('Ctrl Pts',(0.779109323683612,-0.232742381310829,
0.657208095763053));
#12932=CARTESIAN_POINT('Ctrl Pts',(0.750552691816206,-0.244234834628584,
0.68964083160521));
#12933=CARTESIAN_POINT('Ctrl Pts',(0.735185187071673,-0.246942143572133,
0.705971972091755));
#12934=CARTESIAN_POINT('Ctrl Pts',(0.705971972091754,-0.246942143572133,
0.735185187071673));
#12935=CARTESIAN_POINT('Ctrl Pts',(0.689640831605209,-0.244234834628584,
0.750552691816206));
#12936=CARTESIAN_POINT('Ctrl Pts',(0.657208095763052,-0.232742381310829,
0.779109323683612));
#12937=CARTESIAN_POINT('Ctrl Pts',(0.641117951819998,-0.223955109275652,
0.792310597819928));
#12938=CARTESIAN_POINT('Ctrl Pts',(0.609616703125487,-0.201072148666545,
0.816896541396382));
#12939=CARTESIAN_POINT('Ctrl Pts',(0.590422647829571,-0.181890537957858,
0.830754510485544));
#12940=CARTESIAN_POINT('Ctrl Pts',(0.560922177770135,-0.141695629206858,
0.850993704737257));
#12941=CARTESIAN_POINT('Ctrl Pts',(0.547089171823309,-0.115492077056649,
0.859812944202861));
#12942=CARTESIAN_POINT('Ctrl Pts',(0.533674141594226,-0.0742967091364491,
0.868149331745852));
#12943=CARTESIAN_POINT('Ctrl Pts',(0.530395067942936,-0.0609922781173483,
0.870146645090731));
#12944=CARTESIAN_POINT('Ctrl Pts',(0.528110872004958,-0.0476300000000001,
0.871530771444223));
#12945=CARTESIAN_POINT('Origin',(0.707106781186547,-0.04763,0.707106781186548));
#12946=CARTESIAN_POINT('Origin',(0.,-0.166705,0.));
#12947=CARTESIAN_POINT('',(0.242834539687906,-0.04763,0.989696097314));
#12948=CARTESIAN_POINT('Origin',(0.,-0.04763,0.));
#12949=CARTESIAN_POINT('',(-0.242834539687907,-0.04763,0.989696097314));
#12950=CARTESIAN_POINT('Ctrl Pts',(0.242834539687906,-0.04763,0.989696097314));
#12951=CARTESIAN_POINT('Ctrl Pts',(0.24024064412003,-0.0609922781173483,
0.990332542620729));
#12952=CARTESIAN_POINT('Ctrl Pts',(0.236509675094874,-0.0742967091364492,
0.991238884025248));
#12953=CARTESIAN_POINT('Ctrl Pts',(0.221129100087819,-0.115492077056649,
0.994830026707808));
#12954=CARTESIAN_POINT('Ctrl Pts',(0.205111543747588,-0.141695629206859,
0.998375294985966));
#12955=CARTESIAN_POINT('Ctrl Pts',(0.169940289819232,-0.181890537957859,
1.00492400591205));
#12956=CARTESIAN_POINT('Ctrl Pts',(0.1465689792446,-0.201072148666545,1.00869718865384));
#12957=CARTESIAN_POINT('Ctrl Pts',(0.106909345252087,-0.223955109275652,
1.01358704779679));
#12958=CARTESIAN_POINT('Ctrl Pts',(0.0861971848975941,-0.232742381310829,
1.0156297872271));
#12959=CARTESIAN_POINT('Ctrl Pts',(0.0430711894098822,-0.244234834628584,
1.01837060663223));
#12960=CARTESIAN_POINT('Ctrl Pts',(0.0206568624125605,-0.246942143572133,
1.019052));
#12961=CARTESIAN_POINT('Ctrl Pts',(-0.0206568624125608,-0.246942143572133,
1.019052));
#12962=CARTESIAN_POINT('Ctrl Pts',(-0.0430711894098825,-0.244234834628584,
1.01837060663223));
#12963=CARTESIAN_POINT('Ctrl Pts',(-0.0861971848975943,-0.232742381310829,
1.0156297872271));
#12964=CARTESIAN_POINT('Ctrl Pts',(-0.106909345252088,-0.223955109275652,
1.01358704779679));
#12965=CARTESIAN_POINT('Ctrl Pts',(-0.1465689792446,-0.201072148666545,
1.00869718865384));
#12966=CARTESIAN_POINT('Ctrl Pts',(-0.169940289819232,-0.181890537957859,
1.00492400591205));
#12967=CARTESIAN_POINT('Ctrl Pts',(-0.205111543747588,-0.141695629206859,
0.998375294985966));
#12968=CARTESIAN_POINT('Ctrl Pts',(-0.221129100087819,-0.115492077056649,
0.994830026707808));
#12969=CARTESIAN_POINT('Ctrl Pts',(-0.236509675094875,-0.0742967091364493,
0.991238884025248));
#12970=CARTESIAN_POINT('Ctrl Pts',(-0.24024064412003,-0.0609922781173483,
0.990332542620729));
#12971=CARTESIAN_POINT('Ctrl Pts',(-0.242834539687907,-0.04763,0.989696097314));
#12972=CARTESIAN_POINT('',(-0.528110872004959,-0.04763,0.871530771444223));
#12973=CARTESIAN_POINT('Origin',(0.,-0.04763,0.));
#12974=CARTESIAN_POINT('',(-0.871530771444223,-0.04763,0.528110872004958));
#12975=CARTESIAN_POINT('Ctrl Pts',(-0.528110872004958,-0.0476300000000001,
0.871530771444223));
#12976=CARTESIAN_POINT('Ctrl Pts',(-0.530395067942936,-0.0609922781173484,
0.87014664509073));
#12977=CARTESIAN_POINT('Ctrl Pts',(-0.533674141594226,-0.0742967091364493,
0.868149331745851));
#12978=CARTESIAN_POINT('Ctrl Pts',(-0.54708917182331,-0.115492077056649,
0.85981294420286));
#12979=CARTESIAN_POINT('Ctrl Pts',(-0.560922177770136,-0.141695629206859,
0.850993704737257));
#12980=CARTESIAN_POINT('Ctrl Pts',(-0.590422647829571,-0.181890537957859,
0.830754510485543));
#12981=CARTESIAN_POINT('Ctrl Pts',(-0.609616703125488,-0.201072148666545,
0.816896541396381));
#12982=CARTESIAN_POINT('Ctrl Pts',(-0.641117951819998,-0.223955109275652,
0.792310597819928));
#12983=CARTESIAN_POINT('Ctrl Pts',(-0.657208095763053,-0.232742381310829,
0.779109323683611));
#12984=CARTESIAN_POINT('Ctrl Pts',(-0.68964083160521,-0.244234834628584,
0.750552691816205));
#12985=CARTESIAN_POINT('Ctrl Pts',(-0.705971972091755,-0.246942143572133,
0.735185187071673));
#12986=CARTESIAN_POINT('Ctrl Pts',(-0.735185187071673,-0.246942143572133,
0.705971972091754));
#12987=CARTESIAN_POINT('Ctrl Pts',(-0.750552691816206,-0.244234834628584,
0.689640831605209));
#12988=CARTESIAN_POINT('Ctrl Pts',(-0.779109323683612,-0.232742381310829,
0.657208095763052));
#12989=CARTESIAN_POINT('Ctrl Pts',(-0.792310597819928,-0.223955109275652,
0.641117951819998));
#12990=CARTESIAN_POINT('Ctrl Pts',(-0.816896541396382,-0.201072148666545,
0.609616703125487));
#12991=CARTESIAN_POINT('Ctrl Pts',(-0.830754510485544,-0.181890537957858,
0.590422647829571));
#12992=CARTESIAN_POINT('Ctrl Pts',(-0.850993704737257,-0.141695629206858,
0.560922177770135));
#12993=CARTESIAN_POINT('Ctrl Pts',(-0.859812944202861,-0.115492077056649,
0.547089171823309));
#12994=CARTESIAN_POINT('Ctrl Pts',(-0.868149331745852,-0.0742967091364491,
0.533674141594226));
#12995=CARTESIAN_POINT('Ctrl Pts',(-0.870146645090731,-0.0609922781173483,
0.530395067942936));
#12996=CARTESIAN_POINT('Ctrl Pts',(-0.871530771444223,-0.04763,0.528110872004958));
#12997=CARTESIAN_POINT('',(-0.989696097314,-0.04763,0.242834539687906));
#12998=CARTESIAN_POINT('Origin',(0.,-0.04763,0.));
#12999=CARTESIAN_POINT('',(-1.019052,-0.246942143572133,1.248489836334E-16));
#13000=CARTESIAN_POINT('Ctrl Pts',(-0.989696097314,-0.04763,0.242834539687906));
#13001=CARTESIAN_POINT('Ctrl Pts',(-0.990332542620729,-0.0609922781173483,
0.24024064412003));
#13002=CARTESIAN_POINT('Ctrl Pts',(-0.991238884025248,-0.0742967091364492,
0.236509675094874));
#13003=CARTESIAN_POINT('Ctrl Pts',(-0.994830026707808,-0.115492077056649,
0.221129100087819));
#13004=CARTESIAN_POINT('Ctrl Pts',(-0.998375294985966,-0.141695629206859,
0.205111543747588));
#13005=CARTESIAN_POINT('Ctrl Pts',(-1.00492400591205,-0.181890537957859,
0.169940289819232));
#13006=CARTESIAN_POINT('Ctrl Pts',(-1.00869718865384,-0.201072148666545,
0.1465689792446));
#13007=CARTESIAN_POINT('Ctrl Pts',(-1.01358704779679,-0.223955109275652,
0.106909345252088));
#13008=CARTESIAN_POINT('Ctrl Pts',(-1.0156297872271,-0.232742381310829,
0.0861971848975944));
#13009=CARTESIAN_POINT('Ctrl Pts',(-1.01837060663223,-0.244234834628584,
0.0430711894098825));
#13010=CARTESIAN_POINT('Ctrl Pts',(-1.019052,-0.246942143572133,0.0206568624125608));
#13011=CARTESIAN_POINT('Ctrl Pts',(-1.019052,-0.246942143572133,1.2490009027033E-16));
#13012=CARTESIAN_POINT('',(-1.019052,-0.28578,1.24797876996471E-16));
#13013=CARTESIAN_POINT('',(-1.019052,-0.166705,1.24797876996471E-16));
#13014=CARTESIAN_POINT('Origin',(0.,-0.28578,0.));
#13015=CARTESIAN_POINT('',(-0.989696097314,-0.04763,-0.242834539687906));
#13016=CARTESIAN_POINT('Ctrl Pts',(-1.019052,-0.246942143572133,1.2490009027033E-16));
#13017=CARTESIAN_POINT('Ctrl Pts',(-1.019052,-0.246942143572133,-0.0206568624125605));
#13018=CARTESIAN_POINT('Ctrl Pts',(-1.01837060663223,-0.244234834628584,
-0.0430711894098822));
#13019=CARTESIAN_POINT('Ctrl Pts',(-1.0156297872271,-0.232742381310829,
-0.0861971848975941));
#13020=CARTESIAN_POINT('Ctrl Pts',(-1.01358704779679,-0.223955109275652,
-0.106909345252087));
#13021=CARTESIAN_POINT('Ctrl Pts',(-1.00869718865384,-0.201072148666546,
-0.1465689792446));
#13022=CARTESIAN_POINT('Ctrl Pts',(-1.00492400591205,-0.181890537957859,
-0.169940289819232));
#13023=CARTESIAN_POINT('Ctrl Pts',(-0.998375294985966,-0.141695629206859,
-0.205111543747588));
#13024=CARTESIAN_POINT('Ctrl Pts',(-0.994830026707808,-0.11549207705665,
-0.221129100087819));
#13025=CARTESIAN_POINT('Ctrl Pts',(-0.991238884025248,-0.0742967091364495,
-0.236509675094874));
#13026=CARTESIAN_POINT('Ctrl Pts',(-0.990332542620729,-0.0609922781173484,
-0.24024064412003));
#13027=CARTESIAN_POINT('Ctrl Pts',(-0.989696097314,-0.0476300000000001,
-0.242834539687907));
#13028=CARTESIAN_POINT('',(-0.871530771444223,-0.04763,-0.528110872004958));
#13029=CARTESIAN_POINT('Origin',(0.,-0.04763,0.));
#13030=CARTESIAN_POINT('',(-0.528110872004958,-0.04763,-0.871530771444223));
#13031=CARTESIAN_POINT('Ctrl Pts',(-0.871530771444223,-0.0476300000000001,
-0.528110872004958));
#13032=CARTESIAN_POINT('Ctrl Pts',(-0.87014664509073,-0.0609922781173484,
-0.530395067942936));
#13033=CARTESIAN_POINT('Ctrl Pts',(-0.868149331745851,-0.0742967091364494,
-0.533674141594226));
#13034=CARTESIAN_POINT('Ctrl Pts',(-0.85981294420286,-0.115492077056649,
-0.54708917182331));
#13035=CARTESIAN_POINT('Ctrl Pts',(-0.850993704737257,-0.141695629206859,
-0.560922177770136));
#13036=CARTESIAN_POINT('Ctrl Pts',(-0.830754510485543,-0.181890537957859,
-0.590422647829571));
#13037=CARTESIAN_POINT('Ctrl Pts',(-0.816896541396381,-0.201072148666546,
-0.609616703125488));
#13038=CARTESIAN_POINT('Ctrl Pts',(-0.792310597819928,-0.223955109275652,
-0.641117951819999));
#13039=CARTESIAN_POINT('Ctrl Pts',(-0.779109323683611,-0.232742381310829,
-0.657208095763053));
#13040=CARTESIAN_POINT('Ctrl Pts',(-0.750552691816205,-0.244234834628584,
-0.68964083160521));
#13041=CARTESIAN_POINT('Ctrl Pts',(-0.735185187071673,-0.246942143572133,
-0.705971972091755));
#13042=CARTESIAN_POINT('Ctrl Pts',(-0.705971972091754,-0.246942143572133,
-0.735185187071673));
#13043=CARTESIAN_POINT('Ctrl Pts',(-0.68964083160521,-0.244234834628584,
-0.750552691816206));
#13044=CARTESIAN_POINT('Ctrl Pts',(-0.657208095763052,-0.232742381310829,
-0.779109323683612));
#13045=CARTESIAN_POINT('Ctrl Pts',(-0.641117951819998,-0.223955109275652,
-0.792310597819928));
#13046=CARTESIAN_POINT('Ctrl Pts',(-0.609616703125488,-0.201072148666545,
-0.816896541396381));
#13047=CARTESIAN_POINT('Ctrl Pts',(-0.590422647829571,-0.181890537957859,
-0.830754510485543));
#13048=CARTESIAN_POINT('Ctrl Pts',(-0.560922177770136,-0.141695629206859,
-0.850993704737257));
#13049=CARTESIAN_POINT('Ctrl Pts',(-0.54708917182331,-0.115492077056649,
-0.85981294420286));
#13050=CARTESIAN_POINT('Ctrl Pts',(-0.533674141594226,-0.0742967091364494,
-0.868149331745852));
#13051=CARTESIAN_POINT('Ctrl Pts',(-0.530395067942936,-0.0609922781173484,
-0.870146645090731));
#13052=CARTESIAN_POINT('Ctrl Pts',(-0.528110872004958,-0.0476300000000001,
-0.871530771444223));
#13053=CARTESIAN_POINT('',(-0.242834539687906,-0.04763,-0.989696097314));
#13054=CARTESIAN_POINT('Origin',(0.,-0.04763,0.));
#13055=CARTESIAN_POINT('',(0.242834539687906,-0.04763,-0.989696097314));
#13056=CARTESIAN_POINT('Ctrl Pts',(-0.242834539687907,-0.04763,-0.989696097314));
#13057=CARTESIAN_POINT('Ctrl Pts',(-0.24024064412003,-0.0609922781173483,
-0.990332542620729));
#13058=CARTESIAN_POINT('Ctrl Pts',(-0.236509675094874,-0.0742967091364493,
-0.991238884025248));
#13059=CARTESIAN_POINT('Ctrl Pts',(-0.221129100087819,-0.115492077056649,
-0.994830026707808));
#13060=CARTESIAN_POINT('Ctrl Pts',(-0.205111543747588,-0.141695629206859,
-0.998375294985966));
#13061=CARTESIAN_POINT('Ctrl Pts',(-0.169940289819232,-0.181890537957859,
-1.00492400591205));
#13062=CARTESIAN_POINT('Ctrl Pts',(-0.1465689792446,-0.201072148666545,
-1.00869718865384));
#13063=CARTESIAN_POINT('Ctrl Pts',(-0.106909345252087,-0.223955109275652,
-1.01358704779679));
#13064=CARTESIAN_POINT('Ctrl Pts',(-0.0861971848975942,-0.232742381310829,
-1.0156297872271));
#13065=CARTESIAN_POINT('Ctrl Pts',(-0.0430711894098823,-0.244234834628584,
-1.01837060663223));
#13066=CARTESIAN_POINT('Ctrl Pts',(-0.0206568624125606,-0.246942143572133,
-1.019052));
#13067=CARTESIAN_POINT('Ctrl Pts',(0.0206568624125607,-0.246942143572133,
-1.019052));
#13068=CARTESIAN_POINT('Ctrl Pts',(0.0430711894098824,-0.244234834628584,
-1.01837060663223));
#13069=CARTESIAN_POINT('Ctrl Pts',(0.0861971848975943,-0.232742381310829,
-1.0156297872271));
#13070=CARTESIAN_POINT('Ctrl Pts',(0.106909345252088,-0.223955109275652,
-1.01358704779679));
#13071=CARTESIAN_POINT('Ctrl Pts',(0.1465689792446,-0.201072148666545,-1.00869718865384));
#13072=CARTESIAN_POINT('Ctrl Pts',(0.169940289819232,-0.181890537957859,
-1.00492400591205));
#13073=CARTESIAN_POINT('Ctrl Pts',(0.205111543747588,-0.141695629206859,
-0.998375294985966));
#13074=CARTESIAN_POINT('Ctrl Pts',(0.221129100087819,-0.115492077056649,
-0.994830026707808));
#13075=CARTESIAN_POINT('Ctrl Pts',(0.236509675094874,-0.0742967091364493,
-0.991238884025248));
#13076=CARTESIAN_POINT('Ctrl Pts',(0.24024064412003,-0.0609922781173484,
-0.990332542620729));
#13077=CARTESIAN_POINT('Ctrl Pts',(0.242834539687907,-0.04763,-0.989696097314));
#13078=CARTESIAN_POINT('',(0.528110872004958,-0.04763,-0.871530771444223));
#13079=CARTESIAN_POINT('Origin',(0.,-0.04763,0.));
#13080=CARTESIAN_POINT('',(0.871530771444223,-0.04763,-0.528110872004958));
#13081=CARTESIAN_POINT('Ctrl Pts',(0.528110872004958,-0.0476300000000001,
-0.871530771444223));
#13082=CARTESIAN_POINT('Ctrl Pts',(0.530395067942936,-0.0609922781173484,
-0.870146645090731));
#13083=CARTESIAN_POINT('Ctrl Pts',(0.533674141594226,-0.0742967091364493,
-0.868149331745851));
#13084=CARTESIAN_POINT('Ctrl Pts',(0.54708917182331,-0.115492077056649,
-0.85981294420286));
#13085=CARTESIAN_POINT('Ctrl Pts',(0.560922177770136,-0.141695629206859,
-0.850993704737257));
#13086=CARTESIAN_POINT('Ctrl Pts',(0.590422647829571,-0.181890537957859,
-0.830754510485543));
#13087=CARTESIAN_POINT('Ctrl Pts',(0.609616703125488,-0.201072148666545,
-0.816896541396381));
#13088=CARTESIAN_POINT('Ctrl Pts',(0.641117951819998,-0.223955109275652,
-0.792310597819928));
#13089=CARTESIAN_POINT('Ctrl Pts',(0.657208095763053,-0.232742381310829,
-0.779109323683612));
#13090=CARTESIAN_POINT('Ctrl Pts',(0.68964083160521,-0.244234834628584,
-0.750552691816206));
#13091=CARTESIAN_POINT('Ctrl Pts',(0.705971972091755,-0.246942143572133,
-0.735185187071673));
#13092=CARTESIAN_POINT('Ctrl Pts',(0.735185187071673,-0.246942143572133,
-0.705971972091754));
#13093=CARTESIAN_POINT('Ctrl Pts',(0.750552691816206,-0.244234834628584,
-0.68964083160521));
#13094=CARTESIAN_POINT('Ctrl Pts',(0.779109323683612,-0.232742381310829,
-0.657208095763053));
#13095=CARTESIAN_POINT('Ctrl Pts',(0.792310597819928,-0.223955109275652,
-0.641117951819998));
#13096=CARTESIAN_POINT('Ctrl Pts',(0.816896541396381,-0.201072148666545,
-0.609616703125488));
#13097=CARTESIAN_POINT('Ctrl Pts',(0.830754510485543,-0.181890537957859,
-0.590422647829571));
#13098=CARTESIAN_POINT('Ctrl Pts',(0.850993704737257,-0.141695629206859,
-0.560922177770136));
#13099=CARTESIAN_POINT('Ctrl Pts',(0.85981294420286,-0.115492077056649,
-0.54708917182331));
#13100=CARTESIAN_POINT('Ctrl Pts',(0.868149331745851,-0.0742967091364493,
-0.533674141594226));
#13101=CARTESIAN_POINT('Ctrl Pts',(0.870146645090731,-0.0609922781173484,
-0.530395067942936));
#13102=CARTESIAN_POINT('Ctrl Pts',(0.871530771444223,-0.0476300000000001,
-0.528110872004958));
#13103=CARTESIAN_POINT('',(0.989696097314,-0.04763,-0.242834539687906));
#13104=CARTESIAN_POINT('Origin',(0.,-0.04763,0.));
#13105=CARTESIAN_POINT('',(0.989696097314,-0.04763,0.242834539687906));
#13106=CARTESIAN_POINT('Ctrl Pts',(0.989696097314,-0.04763,-0.242834539687907));
#13107=CARTESIAN_POINT('Ctrl Pts',(0.990332542620729,-0.0609922781173483,
-0.24024064412003));
#13108=CARTESIAN_POINT('Ctrl Pts',(0.991238884025248,-0.0742967091364493,
-0.236509675094874));
#13109=CARTESIAN_POINT('Ctrl Pts',(0.994830026707808,-0.115492077056649,
-0.221129100087819));
#13110=CARTESIAN_POINT('Ctrl Pts',(0.998375294985966,-0.141695629206859,
-0.205111543747588));
#13111=CARTESIAN_POINT('Ctrl Pts',(1.00492400591205,-0.181890537957859,
-0.169940289819232));
#13112=CARTESIAN_POINT('Ctrl Pts',(1.00869718865384,-0.201072148666545,
-0.1465689792446));
#13113=CARTESIAN_POINT('Ctrl Pts',(1.01358704779679,-0.223955109275652,
-0.106909345252087));
#13114=CARTESIAN_POINT('Ctrl Pts',(1.0156297872271,-0.232742381310829,-0.0861971848975942));
#13115=CARTESIAN_POINT('Ctrl Pts',(1.01837060663223,-0.244234834628584,
-0.0430711894098823));
#13116=CARTESIAN_POINT('Ctrl Pts',(1.019052,-0.246942143572133,-0.0206568624125607));
#13117=CARTESIAN_POINT('Ctrl Pts',(1.019052,-0.246942143572133,0.0206568624125607));
#13118=CARTESIAN_POINT('Ctrl Pts',(1.01837060663223,-0.244234834628584,
0.0430711894098823));
#13119=CARTESIAN_POINT('Ctrl Pts',(1.0156297872271,-0.232742381310829,0.0861971848975942));
#13120=CARTESIAN_POINT('Ctrl Pts',(1.01358704779679,-0.223955109275652,
0.106909345252087));
#13121=CARTESIAN_POINT('Ctrl Pts',(1.00869718865384,-0.201072148666545,
0.1465689792446));
#13122=CARTESIAN_POINT('Ctrl Pts',(1.00492400591205,-0.181890537957859,
0.169940289819232));
#13123=CARTESIAN_POINT('Ctrl Pts',(0.998375294985966,-0.141695629206859,
0.205111543747588));
#13124=CARTESIAN_POINT('Ctrl Pts',(0.994830026707808,-0.115492077056649,
0.221129100087819));
#13125=CARTESIAN_POINT('Ctrl Pts',(0.991238884025248,-0.0742967091364492,
0.236509675094874));
#13126=CARTESIAN_POINT('Ctrl Pts',(0.990332542620729,-0.0609922781173483,
0.24024064412003));
#13127=CARTESIAN_POINT('Ctrl Pts',(0.989696097314,-0.04763,0.242834539687907));
#13128=CARTESIAN_POINT('Origin',(0.,-0.04763,0.));
#13129=CARTESIAN_POINT('Origin',(0.,-0.04763,0.));
#13130=CARTESIAN_POINT('',(0.238183666596899,-0.04763,0.951592097314));
#13131=CARTESIAN_POINT('Origin',(0.,-0.04763,0.));
#13132=CARTESIAN_POINT('Origin',(-1.94289029309402E-16,-0.04763,1.));
#13133=CARTESIAN_POINT('Origin',(-1.94289029309402E-16,0.,1.));
#13134=CARTESIAN_POINT('',(-0.2381836665969,-0.04763,0.951592097314));
#13135=CARTESIAN_POINT('Ctrl Pts',(-0.238183666596899,-0.0476299999999999,
0.951592097314));
#13136=CARTESIAN_POINT('Ctrl Pts',(-0.233157223576062,-0.0740444353928835,
0.952850216871763));
#13137=CARTESIAN_POINT('Ctrl Pts',(-0.223801617934946,-0.0999305678883309,
0.955173119738174));
#13138=CARTESIAN_POINT('Ctrl Pts',(-0.199966927975188,-0.142345102874864,
0.960411259488514));
#13139=CARTESIAN_POINT('Ctrl Pts',(-0.1868781821531,-0.159766064500479,
0.963103647174702));
#13140=CARTESIAN_POINT('Ctrl Pts',(-0.15681442133453,-0.190326085855194,
0.968453058988463));
#13141=CARTESIAN_POINT('Ctrl Pts',(-0.139836317888043,-0.203463743702801,
0.971100730005489));
#13142=CARTESIAN_POINT('Ctrl Pts',(-0.104422493053067,-0.224161999508995,
0.975530745318961));
#13143=CARTESIAN_POINT('Ctrl Pts',(-0.0842175114474176,-0.232861760990032,
0.977553872336861));
#13144=CARTESIAN_POINT('Ctrl Pts',(-0.0421062857595701,-0.244251601209411,
0.980270995488453));
#13145=CARTESIAN_POINT('Ctrl Pts',(-0.0201990724523197,-0.246942143572133,
0.980948));
#13146=CARTESIAN_POINT('Ctrl Pts',(0.020199072452319,-0.246942143572133,
0.980948));
#13147=CARTESIAN_POINT('Ctrl Pts',(0.0421062857595694,-0.244251601209411,
0.980270995488454));
#13148=CARTESIAN_POINT('Ctrl Pts',(0.0842175114474169,-0.232861760990032,
0.977553872336861));
#13149=CARTESIAN_POINT('Ctrl Pts',(0.104422493053067,-0.224161999508995,
0.975530745318961));
#13150=CARTESIAN_POINT('Ctrl Pts',(0.139836317888042,-0.203463743702801,
0.971100730005489));
#13151=CARTESIAN_POINT('Ctrl Pts',(0.15681442133453,-0.190326085855194,
0.968453058988463));
#13152=CARTESIAN_POINT('Ctrl Pts',(0.1868781821531,-0.15976606450048,0.963103647174702));
#13153=CARTESIAN_POINT('Ctrl Pts',(0.199966927975188,-0.142345102874864,
0.960411259488514));
#13154=CARTESIAN_POINT('Ctrl Pts',(0.223801617934945,-0.0999305678883309,
0.955173119738174));
#13155=CARTESIAN_POINT('Ctrl Pts',(0.233157223576061,-0.0740444353928835,
0.952850216871763));
#13156=CARTESIAN_POINT('Ctrl Pts',(0.238183666596899,-0.0476299999999999,
0.951592097314));
#13157=CARTESIAN_POINT('Origin',(-1.94289029309402E-16,-0.04763,1.));
#13158=CARTESIAN_POINT('Origin',(0.,-0.04763,0.));
#13159=CARTESIAN_POINT('',(-0.504455939115715,-0.04763,0.841298510752802));
#13160=CARTESIAN_POINT('Origin',(0.,-0.04763,0.));
#13161=CARTESIAN_POINT('Origin',(-0.707106781186548,-0.04763,0.707106781186547));
#13162=CARTESIAN_POINT('Origin',(-0.707106781186548,0.,0.707106781186547));
#13163=CARTESIAN_POINT('',(-0.841298510752802,-0.04763,0.504455939115715));
#13164=CARTESIAN_POINT('Ctrl Pts',(-0.841298510752802,-0.04763,0.504455939115715));
#13165=CARTESIAN_POINT('Ctrl Pts',(-0.838633903678357,-0.0740444353928835,
0.508899795931835));
#13166=CARTESIAN_POINT('Ctrl Pts',(-0.833661031856294,-0.0999305678883309,
0.517157748491652));
#13167=CARTESIAN_POINT('Ctrl Pts',(-0.820511285096538,-0.142345102874864,
0.537715343527944));
#13168=CARTESIAN_POINT('Ctrl Pts',(-0.813159949759,-0.159766064500479,0.548874290046456));
#13169=CARTESIAN_POINT('Ctrl Pts',(-0.795684265985089,-0.190326085855194,
0.573915184558107));
#13170=CARTESIAN_POINT('Ctrl Pts',(-0.78555112003688,-0.203463743702801,
0.587792702767295));
#13171=CARTESIAN_POINT('Ctrl Pts',(-0.763642258217233,-0.224161999508995,
0.615966552324775));
#13172=CARTESIAN_POINT('Ctrl Pts',(-0.750785745543687,-0.232861760990032,
0.631684198665438));
#13173=CARTESIAN_POINT('Ctrl Pts',(-0.722929908501543,-0.244251601209411,
0.663382628119203));
#13174=CARTESIAN_POINT('Ctrl Pts',(-0.707917883896095,-0.246942143572133,
0.679352081686668));
#13175=CARTESIAN_POINT('Ctrl Pts',(-0.679352081686668,-0.246942143572133,
0.707917883896095));
#13176=CARTESIAN_POINT('Ctrl Pts',(-0.663382628119203,-0.244251601209411,
0.722929908501544));
#13177=CARTESIAN_POINT('Ctrl Pts',(-0.631684198665438,-0.232861760990031,
0.750785745543687));
#13178=CARTESIAN_POINT('Ctrl Pts',(-0.615966552324775,-0.224161999508995,
0.763642258217233));
#13179=CARTESIAN_POINT('Ctrl Pts',(-0.587792702767295,-0.203463743702801,
0.78555112003688));
#13180=CARTESIAN_POINT('Ctrl Pts',(-0.573915184558107,-0.190326085855194,
0.795684265985088));
#13181=CARTESIAN_POINT('Ctrl Pts',(-0.548874290046456,-0.159766064500479,
0.813159949759));
#13182=CARTESIAN_POINT('Ctrl Pts',(-0.537715343527944,-0.142345102874864,
0.820511285096538));
#13183=CARTESIAN_POINT('Ctrl Pts',(-0.517157748491652,-0.0999305678883309,
0.833661031856294));
#13184=CARTESIAN_POINT('Ctrl Pts',(-0.508899795931835,-0.0740444353928835,
0.838633903678357));
#13185=CARTESIAN_POINT('Ctrl Pts',(-0.504455939115716,-0.04763,0.841298510752801));
#13186=CARTESIAN_POINT('Origin',(-0.707106781186548,-0.04763,0.707106781186547));
#13187=CARTESIAN_POINT('Origin',(0.,-0.04763,0.));
#13188=CARTESIAN_POINT('',(-0.951592097314,-0.04763,0.238183666596899));
#13189=CARTESIAN_POINT('Origin',(0.,-0.04763,0.));
#13190=CARTESIAN_POINT('Origin',(-1.,-0.04763,-1.11022302462516E-16));
#13191=CARTESIAN_POINT('Origin',(-1.,0.,-1.11022302462516E-16));
#13192=CARTESIAN_POINT('',(-0.951592097314,-0.04763,-0.2381836665969));
#13193=CARTESIAN_POINT('',(-0.980948,-0.246942143572133,1.08514323328844E-18));
#13194=CARTESIAN_POINT('Ctrl Pts',(-0.951592097314,-0.04763,-0.238183666596899));
#13195=CARTESIAN_POINT('Ctrl Pts',(-0.952850216871763,-0.0740444353928835,
-0.233157223576062));
#13196=CARTESIAN_POINT('Ctrl Pts',(-0.955173119738174,-0.0999305678883309,
-0.223801617934946));
#13197=CARTESIAN_POINT('Ctrl Pts',(-0.960411259488514,-0.142345102874864,
-0.199966927975188));
#13198=CARTESIAN_POINT('Ctrl Pts',(-0.963103647174702,-0.159766064500479,
-0.1868781821531));
#13199=CARTESIAN_POINT('Ctrl Pts',(-0.968453058988463,-0.190326085855194,
-0.15681442133453));
#13200=CARTESIAN_POINT('Ctrl Pts',(-0.971100730005489,-0.203463743702801,
-0.139836317888043));
#13201=CARTESIAN_POINT('Ctrl Pts',(-0.975530745318961,-0.224161999508995,
-0.104422493053067));
#13202=CARTESIAN_POINT('Ctrl Pts',(-0.977553872336861,-0.232861760990032,
-0.0842175114474175));
#13203=CARTESIAN_POINT('Ctrl Pts',(-0.980270995488453,-0.244251601209411,
-0.0421062857595699));
#13204=CARTESIAN_POINT('Ctrl Pts',(-0.980948,-0.246942143572133,-0.0201990724523195));
#13205=CARTESIAN_POINT('Ctrl Pts',(-0.980948,-0.246942143572133,-1.17961196366423E-16));
#13206=CARTESIAN_POINT('Origin',(-1.,-0.04763,-1.11022302462516E-16));
#13207=CARTESIAN_POINT('Ctrl Pts',(-0.980948,-0.246942143572133,-1.17961196366423E-16));
#13208=CARTESIAN_POINT('Ctrl Pts',(-0.980948,-0.246942143572133,0.0201990724523192));
#13209=CARTESIAN_POINT('Ctrl Pts',(-0.980270995488453,-0.244251601209411,
0.0421062857595695));
#13210=CARTESIAN_POINT('Ctrl Pts',(-0.977553872336861,-0.232861760990032,
0.0842175114474169));
#13211=CARTESIAN_POINT('Ctrl Pts',(-0.975530745318961,-0.224161999508995,
0.104422493053066));
#13212=CARTESIAN_POINT('Ctrl Pts',(-0.971100730005489,-0.203463743702801,
0.139836317888042));
#13213=CARTESIAN_POINT('Ctrl Pts',(-0.968453058988463,-0.190326085855194,
0.15681442133453));
#13214=CARTESIAN_POINT('Ctrl Pts',(-0.963103647174702,-0.15976606450048,
0.1868781821531));
#13215=CARTESIAN_POINT('Ctrl Pts',(-0.960411259488514,-0.142345102874864,
0.199966927975188));
#13216=CARTESIAN_POINT('Ctrl Pts',(-0.955173119738174,-0.099930567888331,
0.223801617934945));
#13217=CARTESIAN_POINT('Ctrl Pts',(-0.952850216871763,-0.0740444353928835,
0.233157223576061));
#13218=CARTESIAN_POINT('Ctrl Pts',(-0.951592097314,-0.04763,0.238183666596899));
#13219=CARTESIAN_POINT('Origin',(0.,-0.04763,0.));
#13220=CARTESIAN_POINT('',(-0.841298510752802,-0.04763,-0.504455939115715));
#13221=CARTESIAN_POINT('Origin',(0.,-0.04763,0.));
#13222=CARTESIAN_POINT('Origin',(-0.707106781186547,-0.04763,-0.707106781186548));
#13223=CARTESIAN_POINT('Origin',(-0.707106781186547,0.,-0.707106781186548));
#13224=CARTESIAN_POINT('',(-0.504455939115715,-0.04763,-0.841298510752802));
#13225=CARTESIAN_POINT('Ctrl Pts',(-0.504455939115715,-0.04763,-0.841298510752802));
#13226=CARTESIAN_POINT('Ctrl Pts',(-0.508899795931835,-0.0740444353928835,
-0.838633903678357));
#13227=CARTESIAN_POINT('Ctrl Pts',(-0.517157748491652,-0.0999305678883309,
-0.833661031856294));
#13228=CARTESIAN_POINT('Ctrl Pts',(-0.537715343527944,-0.142345102874864,
-0.820511285096538));
#13229=CARTESIAN_POINT('Ctrl Pts',(-0.548874290046456,-0.159766064500479,
-0.813159949759));
#13230=CARTESIAN_POINT('Ctrl Pts',(-0.573915184558107,-0.190326085855194,
-0.795684265985089));
#13231=CARTESIAN_POINT('Ctrl Pts',(-0.587792702767295,-0.203463743702801,
-0.78555112003688));
#13232=CARTESIAN_POINT('Ctrl Pts',(-0.615966552324775,-0.224161999508995,
-0.763642258217233));
#13233=CARTESIAN_POINT('Ctrl Pts',(-0.631684198665438,-0.232861760990032,
-0.750785745543687));
#13234=CARTESIAN_POINT('Ctrl Pts',(-0.663382628119203,-0.244251601209411,
-0.722929908501543));
#13235=CARTESIAN_POINT('Ctrl Pts',(-0.679352081686668,-0.246942143572133,
-0.707917883896095));
#13236=CARTESIAN_POINT('Ctrl Pts',(-0.707917883896095,-0.246942143572133,
-0.679352081686668));
#13237=CARTESIAN_POINT('Ctrl Pts',(-0.722929908501543,-0.244251601209411,
-0.663382628119203));
#13238=CARTESIAN_POINT('Ctrl Pts',(-0.750785745543687,-0.232861760990032,
-0.631684198665439));
#13239=CARTESIAN_POINT('Ctrl Pts',(-0.763642258217232,-0.224161999508995,
-0.615966552324775));
#13240=CARTESIAN_POINT('Ctrl Pts',(-0.78555112003688,-0.203463743702801,
-0.587792702767295));
#13241=CARTESIAN_POINT('Ctrl Pts',(-0.795684265985088,-0.190326085855194,
-0.573915184558107));
#13242=CARTESIAN_POINT('Ctrl Pts',(-0.813159949759,-0.15976606450048,-0.548874290046456));
#13243=CARTESIAN_POINT('Ctrl Pts',(-0.820511285096538,-0.142345102874864,
-0.537715343527944));
#13244=CARTESIAN_POINT('Ctrl Pts',(-0.833661031856294,-0.0999305678883311,
-0.517157748491652));
#13245=CARTESIAN_POINT('Ctrl Pts',(-0.838633903678357,-0.0740444353928836,
-0.508899795931835));
#13246=CARTESIAN_POINT('Ctrl Pts',(-0.841298510752801,-0.04763,-0.504455939115715));
#13247=CARTESIAN_POINT('Origin',(-0.707106781186547,-0.04763,-0.707106781186548));
#13248=CARTESIAN_POINT('Origin',(0.,-0.04763,0.));
#13249=CARTESIAN_POINT('',(-0.238183666596899,-0.04763,-0.951592097314));
#13250=CARTESIAN_POINT('Origin',(0.,-0.04763,0.));
#13251=CARTESIAN_POINT('Origin',(5.55111512312578E-17,-0.04763,-1.));
#13252=CARTESIAN_POINT('Origin',(5.55111512312578E-17,0.,-1.));
#13253=CARTESIAN_POINT('',(0.238183666596899,-0.04763,-0.951592097314));
#13254=CARTESIAN_POINT('Ctrl Pts',(0.238183666596899,-0.04763,-0.951592097314));
#13255=CARTESIAN_POINT('Ctrl Pts',(0.233157223576062,-0.0740444353928835,
-0.952850216871763));
#13256=CARTESIAN_POINT('Ctrl Pts',(0.223801617934946,-0.099930567888331,
-0.955173119738174));
#13257=CARTESIAN_POINT('Ctrl Pts',(0.199966927975188,-0.142345102874864,
-0.960411259488514));
#13258=CARTESIAN_POINT('Ctrl Pts',(0.1868781821531,-0.15976606450048,-0.963103647174702));
#13259=CARTESIAN_POINT('Ctrl Pts',(0.15681442133453,-0.190326085855194,
-0.968453058988463));
#13260=CARTESIAN_POINT('Ctrl Pts',(0.139836317888042,-0.203463743702801,
-0.971100730005489));
#13261=CARTESIAN_POINT('Ctrl Pts',(0.104422493053067,-0.224161999508995,
-0.975530745318961));
#13262=CARTESIAN_POINT('Ctrl Pts',(0.0842175114474173,-0.232861760990032,
-0.977553872336861));
#13263=CARTESIAN_POINT('Ctrl Pts',(0.0421062857595698,-0.244251601209411,
-0.980270995488453));
#13264=CARTESIAN_POINT('Ctrl Pts',(0.0201990724523194,-0.246942143572133,
-0.980948));
#13265=CARTESIAN_POINT('Ctrl Pts',(-0.0201990724523193,-0.246942143572133,
-0.980948));
#13266=CARTESIAN_POINT('Ctrl Pts',(-0.0421062857595697,-0.244251601209411,
-0.980270995488453));
#13267=CARTESIAN_POINT('Ctrl Pts',(-0.0842175114474171,-0.232861760990032,
-0.977553872336861));
#13268=CARTESIAN_POINT('Ctrl Pts',(-0.104422493053067,-0.224161999508995,
-0.975530745318961));
#13269=CARTESIAN_POINT('Ctrl Pts',(-0.139836317888042,-0.203463743702801,
-0.971100730005489));
#13270=CARTESIAN_POINT('Ctrl Pts',(-0.15681442133453,-0.190326085855194,
-0.968453058988463));
#13271=CARTESIAN_POINT('Ctrl Pts',(-0.1868781821531,-0.15976606450048,-0.963103647174702));
#13272=CARTESIAN_POINT('Ctrl Pts',(-0.199966927975188,-0.142345102874864,
-0.960411259488514));
#13273=CARTESIAN_POINT('Ctrl Pts',(-0.223801617934945,-0.099930567888331,
-0.955173119738174));
#13274=CARTESIAN_POINT('Ctrl Pts',(-0.233157223576062,-0.0740444353928835,
-0.952850216871763));
#13275=CARTESIAN_POINT('Ctrl Pts',(-0.238183666596899,-0.0476299999999999,
-0.951592097314));
#13276=CARTESIAN_POINT('Origin',(5.55111512312578E-17,-0.04763,-1.));
#13277=CARTESIAN_POINT('Origin',(0.,-0.04763,0.));
#13278=CARTESIAN_POINT('',(0.504455939115715,-0.04763,-0.841298510752802));
#13279=CARTESIAN_POINT('Origin',(0.,-0.04763,0.));
#13280=CARTESIAN_POINT('Origin',(0.707106781186548,-0.04763,-0.707106781186547));
#13281=CARTESIAN_POINT('Origin',(0.707106781186548,0.,-0.707106781186547));
#13282=CARTESIAN_POINT('',(0.841298510752802,-0.04763,-0.504455939115715));
#13283=CARTESIAN_POINT('Ctrl Pts',(0.841298510752802,-0.04763,-0.504455939115715));
#13284=CARTESIAN_POINT('Ctrl Pts',(0.838633903678357,-0.0740444353928835,
-0.508899795931835));
#13285=CARTESIAN_POINT('Ctrl Pts',(0.833661031856294,-0.0999305678883309,
-0.517157748491652));
#13286=CARTESIAN_POINT('Ctrl Pts',(0.820511285096538,-0.142345102874864,
-0.537715343527944));
#13287=CARTESIAN_POINT('Ctrl Pts',(0.813159949759,-0.159766064500479,-0.548874290046456));
#13288=CARTESIAN_POINT('Ctrl Pts',(0.795684265985088,-0.190326085855194,
-0.573915184558107));
#13289=CARTESIAN_POINT('Ctrl Pts',(0.78555112003688,-0.203463743702801,
-0.587792702767295));
#13290=CARTESIAN_POINT('Ctrl Pts',(0.763642258217233,-0.224161999508995,
-0.615966552324775));
#13291=CARTESIAN_POINT('Ctrl Pts',(0.750785745543687,-0.232861760990032,
-0.631684198665438));
#13292=CARTESIAN_POINT('Ctrl Pts',(0.722929908501543,-0.244251601209411,
-0.663382628119203));
#13293=CARTESIAN_POINT('Ctrl Pts',(0.707917883896095,-0.246942143572133,
-0.679352081686668));
#13294=CARTESIAN_POINT('Ctrl Pts',(0.679352081686668,-0.246942143572133,
-0.707917883896095));
#13295=CARTESIAN_POINT('Ctrl Pts',(0.663382628119203,-0.244251601209411,
-0.722929908501543));
#13296=CARTESIAN_POINT('Ctrl Pts',(0.631684198665438,-0.232861760990032,
-0.750785745543687));
#13297=CARTESIAN_POINT('Ctrl Pts',(0.615966552324775,-0.224161999508995,
-0.763642258217232));
#13298=CARTESIAN_POINT('Ctrl Pts',(0.587792702767295,-0.203463743702801,
-0.78555112003688));
#13299=CARTESIAN_POINT('Ctrl Pts',(0.573915184558107,-0.190326085855194,
-0.795684265985088));
#13300=CARTESIAN_POINT('Ctrl Pts',(0.548874290046456,-0.159766064500479,
-0.813159949759));
#13301=CARTESIAN_POINT('Ctrl Pts',(0.537715343527944,-0.142345102874864,
-0.820511285096538));
#13302=CARTESIAN_POINT('Ctrl Pts',(0.517157748491652,-0.099930567888331,
-0.833661031856294));
#13303=CARTESIAN_POINT('Ctrl Pts',(0.508899795931835,-0.0740444353928835,
-0.838633903678357));
#13304=CARTESIAN_POINT('Ctrl Pts',(0.504455939115715,-0.04763,-0.841298510752801));
#13305=CARTESIAN_POINT('Origin',(0.707106781186548,-0.04763,-0.707106781186547));
#13306=CARTESIAN_POINT('Origin',(0.,-0.166705,0.));
#13307=CARTESIAN_POINT('',(-0.980948,-0.28578,1.20131482833E-16));
#13308=CARTESIAN_POINT('Origin',(0.,-0.28578,0.));
#13309=CARTESIAN_POINT('',(-0.980948,-0.166705,1.20131482833E-16));
#13310=CARTESIAN_POINT('',(0.951592097314,-0.04763,0.238183666596899));
#13311=CARTESIAN_POINT('Origin',(0.,-0.04763,0.));
#13312=CARTESIAN_POINT('',(0.951592097314,-0.04763,-0.238183666596899));
#13313=CARTESIAN_POINT('Ctrl Pts',(0.951592097314,-0.04763,0.238183666596899));
#13314=CARTESIAN_POINT('Ctrl Pts',(0.952850216871763,-0.0740444353928835,
0.233157223576062));
#13315=CARTESIAN_POINT('Ctrl Pts',(0.955173119738174,-0.099930567888331,
0.223801617934945));
#13316=CARTESIAN_POINT('Ctrl Pts',(0.960411259488514,-0.142345102874864,
0.199966927975188));
#13317=CARTESIAN_POINT('Ctrl Pts',(0.963103647174702,-0.15976606450048,
0.1868781821531));
#13318=CARTESIAN_POINT('Ctrl Pts',(0.968453058988463,-0.190326085855194,
0.15681442133453));
#13319=CARTESIAN_POINT('Ctrl Pts',(0.971100730005489,-0.203463743702801,
0.139836317888042));
#13320=CARTESIAN_POINT('Ctrl Pts',(0.975530745318961,-0.224161999508995,
0.104422493053067));
#13321=CARTESIAN_POINT('Ctrl Pts',(0.977553872336861,-0.232861760990032,
0.0842175114474172));
#13322=CARTESIAN_POINT('Ctrl Pts',(0.980270995488453,-0.244251601209411,
0.0421062857595697));
#13323=CARTESIAN_POINT('Ctrl Pts',(0.980948,-0.246942143572133,0.0201990724523194));
#13324=CARTESIAN_POINT('Ctrl Pts',(0.980948,-0.246942143572133,-0.0201990724523194));
#13325=CARTESIAN_POINT('Ctrl Pts',(0.980270995488453,-0.244251601209411,
-0.0421062857595697));
#13326=CARTESIAN_POINT('Ctrl Pts',(0.977553872336861,-0.232861760990032,
-0.0842175114474172));
#13327=CARTESIAN_POINT('Ctrl Pts',(0.975530745318961,-0.224161999508995,
-0.104422493053067));
#13328=CARTESIAN_POINT('Ctrl Pts',(0.971100730005489,-0.203463743702801,
-0.139836317888042));
#13329=CARTESIAN_POINT('Ctrl Pts',(0.968453058988463,-0.190326085855194,
-0.15681442133453));
#13330=CARTESIAN_POINT('Ctrl Pts',(0.963103647174702,-0.15976606450048,
-0.1868781821531));
#13331=CARTESIAN_POINT('Ctrl Pts',(0.960411259488514,-0.142345102874864,
-0.199966927975188));
#13332=CARTESIAN_POINT('Ctrl Pts',(0.955173119738174,-0.099930567888331,
-0.223801617934945));
#13333=CARTESIAN_POINT('Ctrl Pts',(0.952850216871763,-0.0740444353928835,
-0.233157223576062));
#13334=CARTESIAN_POINT('Ctrl Pts',(0.951592097314,-0.0476299999999999,-0.238183666596899));
#13335=CARTESIAN_POINT('Origin',(0.,-0.04763,0.));
#13336=CARTESIAN_POINT('Origin',(0.,-0.04763,0.));
#13337=CARTESIAN_POINT('Origin',(1.,-0.04763,0.));
#13338=CARTESIAN_POINT('Origin',(1.,0.,0.));
#13339=CARTESIAN_POINT('Origin',(1.,-0.04763,0.));
#13340=CARTESIAN_POINT('Origin',(0.,-0.28578,0.));
#13341=CARTESIAN_POINT('Origin',(0.,-0.04763,0.));
#14785=UNCERTAINTY_MEASURE_WITH_UNIT(LENGTH_MEASURE(0.001),#14879,
'DISTANCE_ACCURACY_VALUE',
'Maximum model space distance between geometric entities at asserted c
onnectivities');
#14824=UNCERTAINTY_MEASURE_WITH_UNIT(LENGTH_MEASURE(0.001),#14879,
'DISTANCE_ACCURACY_VALUE',
'Maximum model space distance between geometric entities at asserted c
onnectivities');
#14839=(
GEOMETRIC_REPRESENTATION_CONTEXT(3)
GLOBAL_UNCERTAINTY_ASSIGNED_CONTEXT((#14785))
GLOBAL_UNIT_ASSIGNED_CONTEXT((#14879,#14881,#14882))
REPRESENTATION_CONTEXT('','3D')
);
#14878=(
GEOMETRIC_REPRESENTATION_CONTEXT(3)
GLOBAL_UNCERTAINTY_ASSIGNED_CONTEXT((#14824))
GLOBAL_UNIT_ASSIGNED_CONTEXT((#14879,#14881,#14882))
REPRESENTATION_CONTEXT('','3D')
);
#14879=(
LENGTH_UNIT()
NAMED_UNIT(*)
SI_UNIT(.CENTI.,.METRE.)
);
#14881=(
NAMED_UNIT(*)
PLANE_ANGLE_UNIT()
SI_UNIT($,.RADIAN.)
);
#14882=(
NAMED_UNIT(*)
SI_UNIT($,.STERADIAN.)
SOLID_ANGLE_UNIT()
);
#14897=SHAPE_DEFINITION_REPRESENTATION(#14950,#15082);
#14950=PRODUCT_DEFINITION_SHAPE('',$,#15136);
#15082=SHAPE_REPRESENTATION('',(#8766),#14839);
#15121=PRODUCT_DEFINITION_CONTEXT('part definition',#15282,'design');
#15136=PRODUCT_DEFINITION('Cage','Cage',#15189,#15121);
#15189=PRODUCT_DEFINITION_FORMATION('',$,#15298);
#15282=APPLICATION_CONTEXT(
'Core Data for Automotive Mechanical Design Process');
#15283=PRODUCT_CONTEXT('part definition',#15282,'mechanical');
#15298=PRODUCT('Cage','Cage','Cage',(#15283));
#15400=COLOUR_RGB('Grey',0.48,0.52,0.57);
#15401=FILL_AREA_STYLE_COLOUR('',#15400);
#15402=FILL_AREA_STYLE('',(#15401));
#15403=SURFACE_STYLE_FILL_AREA(#15402);
#15404=SURFACE_SIDE_STYLE('',(#15403));
#15405=SURFACE_STYLE_USAGE(.BOTH.,#15404);
#15406=PRESENTATION_STYLE_ASSIGNMENT((#15405));
ENDSEC;
END-ISO-10303-21;
